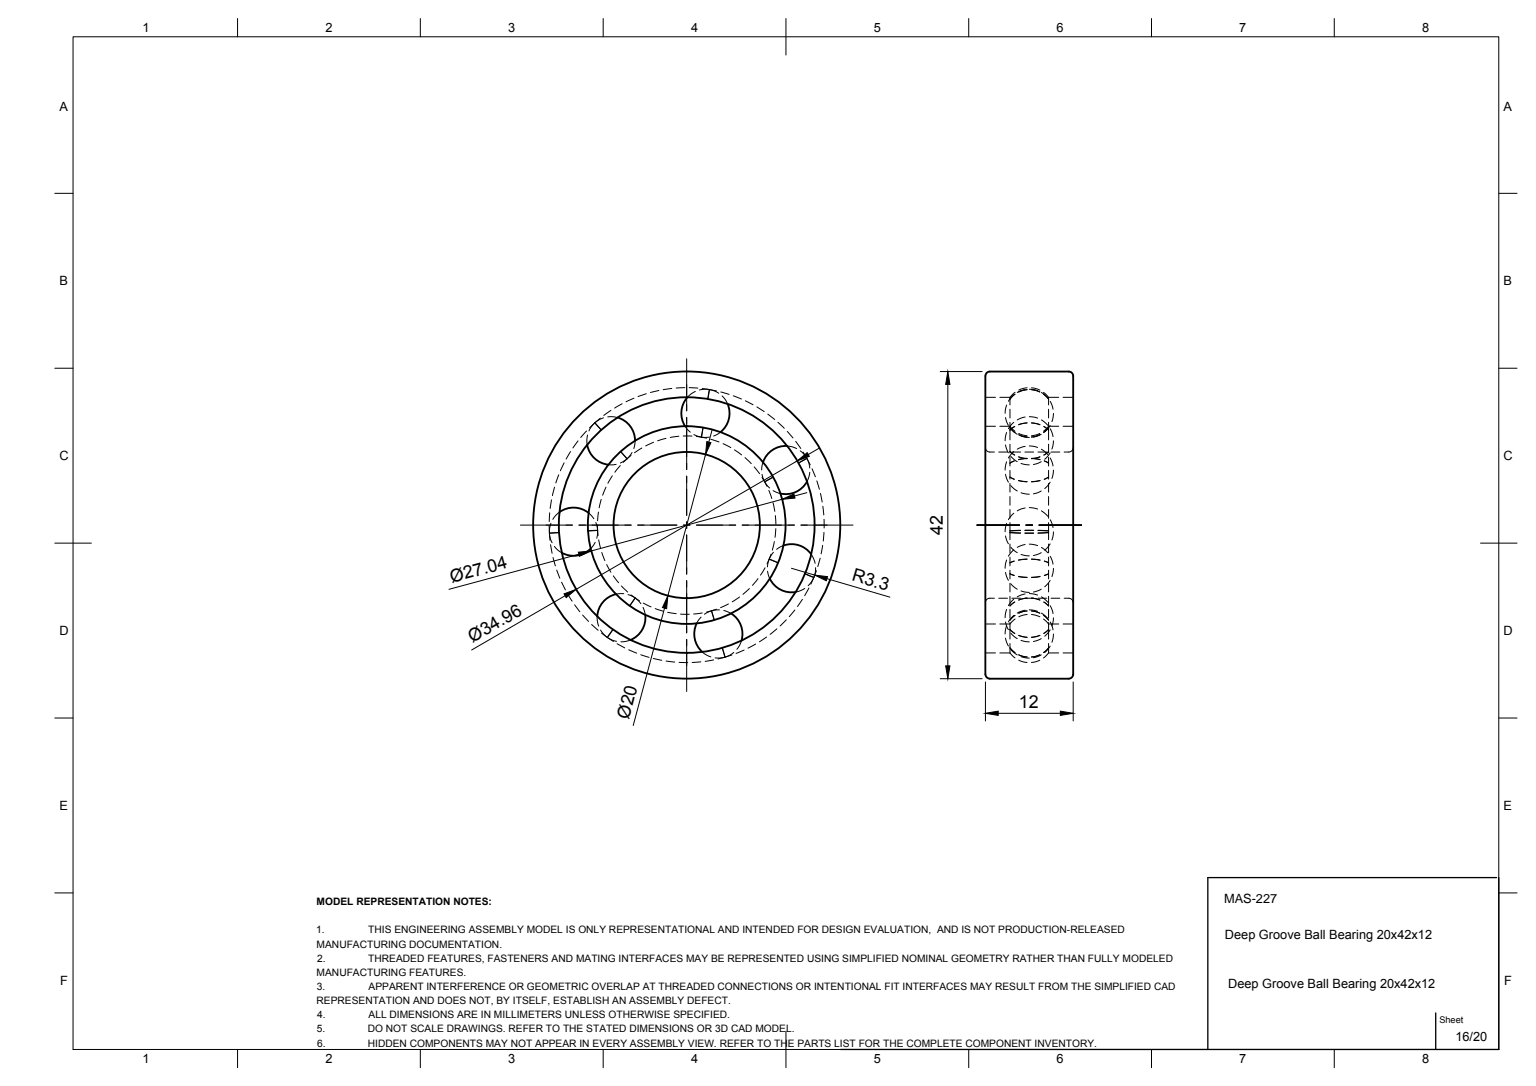
ISO-10303-21;
HEADER;
FILE_DESCRIPTION (('STEP AP214'),
    '1' );
FILE_NAME ( 'Deep Groove Ball Bearing 20x42x12.step', '2026-10-06T08:24:41', ( '' ), ( '' ), 'STEP AP214', 'Unspecified', '' );
FILE_SCHEMA (( 'AUTOMOTIVE_DESIGN' ));
ENDSEC;
DATA;
#17=EDGE_LOOP ( 'NONE', ( #23357, #276 ) ) ;
#28=EDGE_LOOP ( 'NONE', ( #27536, #25941, #6890, #26998 ) ) ;
#30=CARTESIAN_POINT ( 'NONE',  ( -0.5949363243629232079, -0.1357903337134990229, 0.2362204724409449064 ) ) ;
#38=AXIS2_PLACEMENT_3D ( 'NONE', #5001, #26071, #6729 ) ;
#39=CARTESIAN_POINT ( 'NONE',  ( 0.000000000000000000, 0.000000000000000000, 0.06614173228346456601 ) ) ;
#43=CARTESIAN_POINT ( 'NONE',  ( 0.000000000000000000, 0.000000000000000000, 0.2362204724409449064 ) ) ;
#48=ORIENTED_EDGE ( 'NONE', *, *, #8188, .T. ) ;
#58=CARTESIAN_POINT ( 'NONE',  ( 0.4771018889076559244, 0.3804760601893846794, 0.2362204724409449064 ) ) ;
#64=CARTESIAN_POINT ( 'NONE',  ( 0.4157391792961063204, 0.3323952789219082882, 0.1322834645669291320 ) ) ;
#67=CARTESIAN_POINT ( 'NONE',  ( 0.8031496062992127261, 0.000000000000000000, 0.4488188976377953110 ) ) ;
#86=EDGE_CURVE ( 'NONE', #9806, #21006, #24069, .T. ) ;
#87=FACE_BOUND ( 'NONE', #23508, .T. ) ;
#107=ORIENTED_EDGE ( 'NONE', *, *, #20255, .T. ) ;
#109=ADVANCED_FACE ( 'NONE', ( #134 ), #14626, .F. ) ;
#134=FACE_OUTER_BOUND ( 'NONE', #7605, .T. ) ;
#136=CARTESIAN_POINT ( 'NONE',  ( 0.000000000000000000, 0.000000000000000000, 0.2362204724409449064 ) ) ;
#143=CARTESIAN_POINT ( 'NONE',  ( 0.5614173959481695286, 0.4467232815848914962, 0.1601585119481469810 ) ) ;
#153=AXIS2_PLACEMENT_3D ( 'NONE', #12101, #3470, #22847 ) ;
#167=DIRECTION ( 'NONE',  ( 1.000000000000000000, 0.000000000000000000, 0.000000000000000000 ) ) ;
#178=CARTESIAN_POINT ( 'NONE',  ( 0.000000000000000000, 0.000000000000000000, 0.2362204724409449064 ) ) ;
#185=CARTESIAN_POINT ( 'NONE',  ( 0.0007595033562148819414, 0.6881885572739390167, 0.1322834645669291320 ) ) ;
#209=EDGE_CURVE ( 'NONE', #16657, #13154, #17294, .T. ) ;
#219=VECTOR ( 'NONE', #3397, 39.37007874015748143 ) ;
#223=CARTESIAN_POINT ( 'NONE',  ( 0.0005057506112066243896, 0.6881888373222778688, 0.3401591245381555551 ) ) ;
#242=AXIS2_PLACEMENT_3D ( 'NONE', #867, #7637, #22743 ) ;
#257=AXIS2_PLACEMENT_3D ( 'NONE', #24962, #7448, #3195 ) ;
#267=EDGE_CURVE ( 'NONE', #4877, #9806, #20517, .T. ) ;
#269=CARTESIAN_POINT ( 'NONE',  ( 0.3751294191746885609, 0.2999672986753447734, 0.2362204724409446843 ) ) ;
#276=ORIENTED_EDGE ( 'NONE', *, *, #1809, .T. ) ;
#297=CARTESIAN_POINT ( 'NONE',  ( -0.6708219662590964028, -0.1536294932067021612, 0.1322818203437344520 ) ) ;
#299=CARTESIAN_POINT ( 'NONE',  ( -0.5190862322091315262, -0.1177929122753175184, 0.3401574803149606252 ) ) ;
#335=CARTESIAN_POINT ( 'NONE',  ( 0.000000000000000000, 0.000000000000000000, 0.2362204724409449064 ) ) ;
#338=ORIENTED_EDGE ( 'NONE', *, *, #23140, .F. ) ;
#350=CARTESIAN_POINT ( 'NONE',  ( 0.6996455634132897616, -0.1588938903156011662, 0.1601585119484411623 ) ) ;
#389=DIMENSIONAL_EXPONENTS ( 1.000000000000000000, 0.000000000000000000, 0.000000000000000000, 0.000000000000000000, 0.000000000000000000, 0.000000000000000000, 0.000000000000000000 ) ;
#397=B_SPLINE_CURVE_WITH_KNOTS ( 'NONE', 3,
 ( #22454, #26273, #15820, #17525, #20191, #11434, #11714, #3081 ),
 .UNSPECIFIED., .F., .F.,
 ( 4, 2, 2, 4 ),
 ( 0.5000000000000000000, 0.7499999999999997780, 0.8749999999999998890, 1.000000000000000000 ),
 .UNSPECIFIED. ) ;
#401=VERTEX_POINT ( 'NONE', #26015 ) ;
#410=DIRECTION ( 'NONE',  ( 0.000000000000000000, 0.000000000000000000, 1.000000000000000000 ) ) ;
#414=ORIENTED_EDGE ( 'NONE', *, *, #16074, .T. ) ;
#422=CARTESIAN_POINT ( 'NONE',  ( -0.5188388941967637669, -0.1188778293835246053, 0.3401591244667909186 ) ) ;
#423=CIRCLE ( 'NONE', #2649, 0.6881889763779527325 ) ;
#428=ORIENTED_EDGE ( 'NONE', *, *, #19664, .T. ) ;
#432=ORIENTED_EDGE ( 'NONE', *, *, #5914, .T. ) ;
#456=CARTESIAN_POINT ( 'NONE',  ( -0.4684132450478830645, -0.1062614382955276715, 0.2362204724409449619 ) ) ;
#460=CARTESIAN_POINT ( 'NONE',  ( -0.5190862322091315262, -0.1177929122753175184, 0.3401574803149606252 ) ) ;
#462=CARTESIAN_POINT ( 'NONE',  ( 0.4887136534578185310, -0.1122103150229527835, 0.1643955689280507948 ) ) ;
#467=CARTESIAN_POINT ( 'NONE',  ( -0.2981382804007346454, -0.6202561546315846774, 0.1322818203437346463 ) ) ;
#489=CIRCLE ( 'NONE', #20321, 0.5322834645669292097 ) ;
#491=ADVANCED_FACE ( 'NONE', ( #21504 ), #18663, .F. ) ;
#492=FACE_BOUND ( 'NONE', #4958, .T. ) ;
#506=ORIENTED_EDGE ( 'NONE', *, *, #4372, .T. ) ;
#523=EDGE_LOOP ( 'NONE', ( #21704, #21460, #12292, #1622, #7292, #18239 ) ) ;
#531=ORIENTED_EDGE ( 'NONE', *, *, #2877, .F. ) ;
#536=CIRCLE ( 'NONE', #16320, 0.3937007874015748254 ) ;
#543=CARTESIAN_POINT ( 'NONE',  ( -0.0006620872580281702332, 0.5229309616561139684, 0.3331434174598592590 ) ) ;
#548=CARTESIAN_POINT ( 'NONE',  ( 0.0006679551606482677165, 0.5322830454629158270, 0.1322834645669291320 ) ) ;
#554=ORIENTED_EDGE ( 'NONE', *, *, #13765, .T. ) ;
#565=ADVANCED_FACE ( 'NONE', ( #2546 ), #3319, .F. ) ;
#570=CARTESIAN_POINT ( 'NONE',  ( 0.3105958729527036888, -0.6467467715322953170, 0.3122824329341910010 ) ) ;
#577=CARTESIAN_POINT ( 'NONE',  ( 0.000000000000000000, 0.000000000000000000, 0.2362204724409449064 ) ) ;
#598=CARTESIAN_POINT ( 'NONE',  ( 0.6996455634117477729, -0.1588938903152396498, 0.3122824329354899064 ) ) ;
#600=CIRCLE ( 'NONE', #12333, 0.8267716535433071723 ) ;
#618=CARTESIAN_POINT ( 'NONE',  ( -0.0005057506112066828281, 0.6881888373222776467, 0.3401591245381555551 ) ) ;
#619=CARTESIAN_POINT ( 'NONE',  ( 0.2988215684304370012, -0.6199272547993012195, 0.3401599409343967761 ) ) ;
#626=DIRECTION ( 'NONE',  ( 0.000000000000000000, 1.000000000000000000, 0.000000000000000000 ) ) ;
#644=ORIENTED_EDGE ( 'NONE', *, *, #7697, .T. ) ;
#682=SPHERICAL_SURFACE ( 'NONE', #15113, 0.1299232283464566984 ) ;
#695=ORIENTED_EDGE ( 'NONE', *, *, #25428, .F. ) ;
#699=CARTESIAN_POINT ( 'NONE',  ( 0.3759206409296169116, 0.2989751379763687655, 0.2362204724409450174 ) ) ;
#708=FACE_OUTER_BOUND ( 'NONE', #15095, .T. ) ;
#712=DIRECTION ( 'NONE',  ( 0.000000000000000000, -1.000000000000000000, 0.000000000000000000 ) ) ;
#728=CARTESIAN_POINT ( 'NONE',  ( 0.5385210225480960844, 0.4284847435812472183, 0.1322834645669291320 ) ) ;
#739=CARTESIAN_POINT ( 'NONE',  ( 0.000000000000000000, 0.000000000000000000, -1.092739370078740131E-17 ) ) ;
#758=FACE_BOUND ( 'NONE', #21251, .T. ) ;
#768=CARTESIAN_POINT ( 'NONE',  ( 0.0006679551606482677165, 0.5322830454629158270, 0.3401574803149606252 ) ) ;
#793=ORIENTED_EDGE ( 'NONE', *, *, #18272, .F. ) ;
#809=PLANE ( 'NONE',  #6198 ) ;
#819=CARTESIAN_POINT ( 'NONE',  ( -0.2303471512294322787, -0.4798602677570401598, 0.1322834645669291320 ) ) ;
#842=CARTESIAN_POINT ( 'NONE',  ( 0.4092566936341573980, 0.3255244810069335970, 0.3331434174606269227 ) ) ;
#864=CARTESIAN_POINT ( 'NONE',  ( 0.2092582568863658732, -0.4359957531143022202, 0.2715646632236008440 ) ) ;
#867=CARTESIAN_POINT ( 'NONE',  ( 0.000000000000000000, 0.000000000000000000, 0.2362204724409449064 ) ) ;
#874=LINE ( 'NONE', #22052, #17827 ) ;
#883=AXIS2_PLACEMENT_3D ( 'NONE', #21381, #23084, #14476 ) ;
#899=CARTESIAN_POINT ( 'NONE',  ( 0.2315507648392299000, -0.4792806379917101678, 0.1322834645669291320 ) ) ;
#901=EDGE_CURVE ( 'NONE', #11142, #9968, #10681, .T. ) ;
#902=CARTESIAN_POINT ( 'NONE',  ( 0.2307489990847578776, -0.4796672131996535526, 0.1322810039474933141 ) ) ;
#908=ORIENTED_EDGE ( 'NONE', *, *, #10737, .T. ) ;
#910=CARTESIAN_POINT ( 'NONE',  ( 0.4157391792961063204, 0.3323952789219082882, 0.1322834645669291320 ) ) ;
#929=AXIS2_PLACEMENT_3D ( 'NONE', #24250, #9255, #13939 ) ;
#942=ORIENTED_EDGE ( 'NONE', *, *, #7366, .T. ) ;
#956=( GEOMETRIC_REPRESENTATION_CONTEXT ( 3 ) GLOBAL_UNCERTAINTY_ASSIGNED_CONTEXT ( ( #13843 ) ) GLOBAL_UNIT_ASSIGNED_CONTEXT ( ( #21076, #968, #13392 ) ) REPRESENTATION_CONTEXT ( 'NONE', 'WORKASPACE' ) ) ;
#962=CARTESIAN_POINT ( 'NONE',  ( -0.7168072604740280962, -0.1644124225524362104, 0.2763636194370550636 ) ) ;
#967=EDGE_CURVE ( 'NONE', #6542, #17886, #4274, .T. ) ;
#968=( NAMED_UNIT ( * ) PLANE_ANGLE_UNIT ( ) SI_UNIT ( $, .RADIAN. ) ) ;
#972=ORIENTED_EDGE ( 'NONE', *, *, #10601, .F. ) ;
#991=FACE_OUTER_BOUND ( 'NONE', #24406, .T. ) ;
#996=EDGE_LOOP ( 'NONE', ( #23679, #19613, #11944, #25991 ) ) ;
#1016=B_SPLINE_CURVE_WITH_KNOTS ( 'NONE', 3,
 ( #6689, #6828, #4154, #12764, #10638, #19260, #23362, #17146 ),
 .UNSPECIFIED., .F., .F.,
 ( 4, 2, 2, 4 ),
 ( 0.5000000000000000000, 0.7500000000000000000, 0.8749999999999998890, 1.000000000000000000 ),
 .UNSPECIFIED. ) ;
#1017=DIRECTION ( 'NONE',  ( 1.000000000000000000, 0.000000000000000000, 0.000000000000000000 ) ) ;
#1041=DIRECTION ( 'NONE',  ( 0.000000000000000000, -1.000000000000000000, 0.000000000000000000 ) ) ;
#1063=CARTESIAN_POINT ( 'NONE',  ( -0.2274877609455561167, -0.4708572476080006841, 0.1392975274314397494 ) ) ;
#1067=DIRECTION ( 'NONE',  ( -0.2225209339563148925, -0.9749279121818235083, 0.000000000000000000 ) ) ;
#1068=EDGE_CURVE ( 'NONE', #24735, #4219, #15983, .T. ) ;
#1069=EDGE_LOOP ( 'NONE', ( #7141, #12529 ) ) ;
#1077=CARTESIAN_POINT ( 'NONE',  ( 0.4771018889076559244, 0.3804760601893846794, 0.2362204724409449064 ) ) ;
#1094=CARTESIAN_POINT ( 'NONE',  ( 0.000000000000000000, 0.000000000000000000, 0.1322834645669291320 ) ) ;
#1102=AXIS2_PLACEMENT_3D ( 'NONE', #11901, #14175, #1443 ) ;
#1104=CARTESIAN_POINT ( 'NONE',  ( -8.427884271297532088E-17, -0.6881889763779527325, -1.092739370078740131E-17 ) ) ;
#1118=CARTESIAN_POINT ( 'NONE',  ( 0.6708784387195235732, -0.1533826961018693036, 0.3401599409343967761 ) ) ;
#1141=TOROIDAL_SURFACE ( 'NONE', #20078, 0.6102362204724409711, 0.1299212598425196763 ) ;
#1160=ADVANCED_FACE ( 'NONE', ( #25108, #24822 ), #23001, .T. ) ;
#1161=CIRCLE ( 'NONE', #15602, 0.8031496062992127261 ) ;
#1162=ADVANCED_FACE ( 'NONE', ( #9991 ), #18161, .F. ) ;
#1173=CARTESIAN_POINT ( 'NONE',  ( -0.4771018889076559244, 0.3804760601893846794, 0.2362204724409449064 ) ) ;
#1183=DIRECTION ( 'NONE',  ( 0.000000000000000000, 0.000000000000000000, -1.000000000000000000 ) ) ;
#1191=ORIENTED_EDGE ( 'NONE', *, *, #24120, .T. ) ;
#1206=EDGE_LOOP ( 'NONE', ( #20592, #15757, #18634, #4273, #12078, #24003 ) ) ;
#1208=EDGE_CURVE ( 'NONE', #4395, #4877, #8780, .T. ) ;
#1211=DIRECTION ( 'NONE',  ( 1.000000000000000000, 0.000000000000000000, 0.000000000000000000 ) ) ;
#1236=DIRECTION ( 'NONE',  ( 0.000000000000000000, 0.000000000000000000, 1.000000000000000000 ) ) ;
#1237=B_SPLINE_CURVE_WITH_KNOTS ( 'NONE', 3,
 ( #6570, #10655, #1901, #23804, #17029, #25640 ),
 .UNSPECIFIED., .F., .F.,
 ( 4, 2, 4 ),
 ( 1.217380381967464009, 1.219305002860850085, 1.221229623754233939 ),
 .UNSPECIFIED. ) ;
#1243=CARTESIAN_POINT ( 'NONE',  ( -0.7214243740396926174, -0.1654689342655534801, 0.2161412452766471592 ) ) ;
#1261=( GEOMETRIC_REPRESENTATION_CONTEXT ( 3 ) GLOBAL_UNCERTAINTY_ASSIGNED_CONTEXT ( ( #4018 ) ) GLOBAL_UNIT_ASSIGNED_CONTEXT ( ( #20102, #7243, #11487 ) ) REPRESENTATION_CONTEXT ( 'NONE', 'WORKASPACE' ) ) ;
#1281=ORIENTED_EDGE ( 'NONE', *, *, #26449, .F. ) ;
#1291=ORIENTED_EDGE ( 'NONE', *, *, #14066, .F. ) ;
#1300=ORIENTED_EDGE ( 'NONE', *, *, #15873, .F. ) ;
#1307=CARTESIAN_POINT ( 'NONE',  ( -8.427884271297532088E-17, -0.6881889763779527325, 0.06614173228346456601 ) ) ;
#1313=ORIENTED_EDGE ( 'NONE', *, *, #2014, .T. ) ;
#1321=AXIS2_PLACEMENT_3D ( 'NONE', #1328, #3417, #16302 ) ;
#1328=CARTESIAN_POINT ( 'NONE',  ( 0.000000000000000000, 0.000000000000000000, 0.1322834645669291320 ) ) ;
#1334=CARTESIAN_POINT ( 'NONE',  ( -0.4684132450478830645, -0.1062614382955276715, 0.2362204724409449619 ) ) ;
#1347=DIRECTION ( 'NONE',  ( 1.000000000000000000, 0.000000000000000000, 0.000000000000000000 ) ) ;
#1366=EDGE_CURVE ( 'NONE', #18057, #27874, #11501, .T. ) ;
#1385=CARTESIAN_POINT ( 'NONE',  ( 0.2992781133268291316, -0.6197069291944922176, 0.1322834645669291320 ) ) ;
#1386=DIRECTION ( 'NONE',  ( 0.000000000000000000, -1.000000000000000000, 0.000000000000000000 ) ) ;
#1410=EDGE_LOOP ( 'NONE', ( #2496, #1567, #26591, #14884 ) ) ;
#1421=VERTEX_POINT ( 'NONE', #8166 ) ;
#1426=TOROIDAL_SURFACE ( 'NONE', #22181, 0.8031496062992127261, 0.02362204724409448786 ) ;
#1437=CARTESIAN_POINT ( 'NONE',  ( -0.4887136534571460689, -0.1122103150228022234, 0.3080453759528285484 ) ) ;
#1443=DIRECTION ( 'NONE',  ( 0.000000000000000000, 1.000000000000000000, 0.000000000000000000 ) ) ;
#1449=ORIENTED_EDGE ( 'NONE', *, *, #11538, .T. ) ;
#1452=CARTESIAN_POINT ( 'NONE',  ( 0.2078289949484099508, -0.4330237525398077936, 0.2362204724409449619 ) ) ;
#1461=ORIENTED_EDGE ( 'NONE', *, *, #22420, .T. ) ;
#1474=EDGE_CURVE ( 'NONE', #21273, #6542, #24194, .T. ) ;
#1479=CARTESIAN_POINT ( 'NONE',  ( 0.5781866216494347954, 0.4620966632776112304, 0.2562996996002243066 ) ) ;
#1491=ORIENTED_EDGE ( 'NONE', *, *, #6631, .F. ) ;
#1508=TOROIDAL_SURFACE ( 'NONE', #17296, 0.6102362204724409711, 0.1299212598425196763 ) ;
#1515=CARTESIAN_POINT ( 'NONE',  ( 0.000000000000000000, 0.000000000000000000, 0.3401574803149606252 ) ) ;
#1516=AXIS2_PLACEMENT_3D ( 'NONE', #8600, #17220, #167 ) ;
#1523=DIRECTION ( 'NONE',  ( 0.000000000000000000, 0.000000000000000000, 1.000000000000000000 ) ) ;
#1526=EDGE_CURVE ( 'NONE', #23608, #18057, #15118, .T. ) ;
#1527=CARTESIAN_POINT ( 'NONE',  ( 0.000000000000000000, 0.000000000000000000, 0.4062992125984251635 ) ) ;
#1538=EDGE_CURVE ( 'NONE', #8989, #14684, #13758, .T. ) ;
#1539=EDGE_CURVE ( 'NONE', #2213, #9968, #20982, .T. ) ;
#1542=SPHERICAL_SURFACE ( 'NONE', #17946, 0.1299232283464566984 ) ;
#1564=VERTEX_POINT ( 'NONE', #24234 ) ;
#1565=EDGE_CURVE ( 'NONE', #2213, #15981, #2226, .T. ) ;
#1567=ORIENTED_EDGE ( 'NONE', *, *, #26156, .F. ) ;
#1575=CARTESIAN_POINT ( 'NONE',  ( -0.0006679551606482677165, 0.5322830454629158270, 0.3401574803149606252 ) ) ;
#1577=EDGE_LOOP ( 'NONE', ( #3628, #6530 ) ) ;
#1590=CIRCLE ( 'NONE', #2500, 0.02362204724409448092 ) ;
#1608=EDGE_CURVE ( 'NONE', #17836, #10270, #11374, .T. ) ;
#1622=ORIENTED_EDGE ( 'NONE', *, *, #6377, .T. ) ;
#1628=EDGE_CURVE ( 'NONE', #9678, #24310, #22787, .T. ) ;
#1647=B_SPLINE_CURVE_WITH_KNOTS ( 'NONE', 3,
 ( #2295, #10921, #26037, #9470, #11886, #5244 ),
 .UNSPECIFIED., .F., .F.,
 ( 4, 2, 4 ),
 ( 0.4045103800605749922, 0.4064350009536160102, 0.4083596218466570282 ),
 .UNSPECIFIED. ) ;
#1679=DIRECTION ( 'NONE',  ( 0.000000000000000000, 0.000000000000000000, 1.000000000000000000 ) ) ;
#1680=CARTESIAN_POINT ( 'NONE',  ( -0.5385210225480960844, 0.4284847435812472183, 0.1322834645669291320 ) ) ;
#1693=EDGE_CURVE ( 'NONE', #27602, #16511, #21795, .T. ) ;
#1712=CARTESIAN_POINT ( 'NONE',  ( 0.0002221395201541382898, 0.5322834645669292097, 0.1322810039474933141 ) ) ;
#1718=EDGE_CURVE ( 'NONE', #4754, #27858, #20544, .T. ) ;
#1720=EDGE_CURVE ( 'NONE', #27077, #22659, #4736, .T. ) ;
#1730=AXIS2_PLACEMENT_3D ( 'NONE', #1173, #4976, #2977 ) ;
#1732=CIRCLE ( 'NONE', #27448, 0.02362204724409448786 ) ;
#1746=DIRECTION ( 'NONE',  ( 0.000000000000000000, 0.000000000000000000, 1.000000000000000000 ) ) ;
#1755=VERTEX_POINT ( 'NONE', #9920 ) ;
#1762=DIRECTION ( 'NONE',  ( 1.000000000000000000, 0.000000000000000000, 0.000000000000000000 ) ) ;
#1772=AXIS2_PLACEMENT_3D ( 'NONE', #26756, #16030, #5286 ) ;
#1774=AXIS2_PLACEMENT_3D ( 'NONE', #6050, #23287, #16772 ) ;
#1794=AXIS2_PLACEMENT_3D ( 'NONE', #3332, #8026, #8807 ) ;
#1809=EDGE_CURVE ( 'NONE', #18324, #3673, #7442, .T. ) ;
#1814=ORIENTED_EDGE ( 'NONE', *, *, #967, .F. ) ;
#1837=ORIENTED_EDGE ( 'NONE', *, *, #5197, .F. ) ;
#1844=CARTESIAN_POINT ( 'NONE',  ( -0.3062557396300204515, -0.6341756901046630146, 0.1443310008627645136 ) ) ;
#1874=DIRECTION ( 'NONE',  ( 0.6234898018587330393, -0.7818314824680302477, 0.000000000000000000 ) ) ;
#1878=ORIENTED_EDGE ( 'NONE', *, *, #21317, .T. ) ;
#1901=CARTESIAN_POINT ( 'NONE',  ( -0.6708784387195235732, -0.1533826961018689150, 0.3401599409343967761 ) ) ;
#1928=CARTESIAN_POINT ( 'NONE',  ( -0.7171569026305500971, -0.1628805401855070167, 0.2763636194294596948 ) ) ;
#1931=ADVANCED_FACE ( 'NONE', ( #21885, #3056 ), #18165, .T. ) ;
#1942=VERTEX_POINT ( 'NONE', #2521 ) ;
#1963=CARTESIAN_POINT ( 'NONE',  ( -0.6711032387266614441, -0.1523958994813200962, 0.1322834645669291320 ) ) ;
#1971=CLOSED_SHELL ( 'NONE', ( #15948, #15056, #8958, #16202, #10885, #14911, #6900, #2595, #9142, #9759, #11797, #21604, #23526, #3346, #19780, #1160, #17922, #5843, #15313, #9809, #10332, #20220, #565, #12662, #11099, #23134, #1162, #26300, #20891, #109, #23751, #26904, #15516, #491, #12592, #16279, #12320, #22712, #12212, #21149, #4868, #10021, #11378, #13614, #8619, #10786, #4999, #11411, #19167, #7508, #16182, #21953, #18937, #16308, #1931, #10879, #21976, #24048, #23772, #7397, #25804, #17407 ) ) ;
#1974=CARTESIAN_POINT ( 'NONE',  ( 0.3119936278842271316, -0.6460736482368880651, 0.3122824329307916646 ) ) ;
#1978=SPHERICAL_SURFACE ( 'NONE', #5233, 0.1299232283464566984 ) ;
#1997=CARTESIAN_POINT ( 'NONE',  ( 0.000000000000000000, 0.000000000000000000, 0.2362204724409449064 ) ) ;
#2014=EDGE_CURVE ( 'NONE', #22651, #5888, #26397, .T. ) ;
#2016=DIRECTION ( 'NONE',  ( 0.000000000000000000, 0.000000000000000000, -1.000000000000000000 ) ) ;
#2058=AXIS2_PLACEMENT_3D ( 'NONE', #16152, #15733, #24751 ) ;
#2087=ORIENTED_EDGE ( 'NONE', *, *, #5920, .F. ) ;
#2105=CARTESIAN_POINT ( 'NONE',  ( -0.6708784387195275700, -0.1533826961018543433, 0.1322810039474933141 ) ) ;
#2118=CARTESIAN_POINT ( 'NONE',  ( 0.3197948809237959322, -0.6622502000717108706, 0.2763636194327128148 ) ) ;
#2128=CARTESIAN_POINT ( 'NONE',  ( 0.000000000000000000, 0.000000000000000000, -1.092739370078740131E-17 ) ) ;
#2131=CARTESIAN_POINT ( 'NONE',  ( -0.2979095355689177493, -0.6203660015065670663, 0.1322834645669291320 ) ) ;
#2134=CARTESIAN_POINT ( 'NONE',  ( 0.000000000000000000, 0.6881889763779527325, 0.1322810039474933141 ) ) ;
#2167=CARTESIAN_POINT ( 'NONE',  ( 0.000000000000000000, 0.000000000000000000, 0.2362204724409449064 ) ) ;
#2192=CARTESIAN_POINT ( 'NONE',  ( 0.5190862322091315262, -0.1177929122753177127, 0.1322834645669291320 ) ) ;
#2213=VERTEX_POINT ( 'NONE', #10133 ) ;
#2217=AXIS2_PLACEMENT_3D ( 'NONE', #27293, #25163, #7943 ) ;
#2226=B_SPLINE_CURVE_WITH_KNOTS ( 'NONE', 3,
 ( #2337, #9236, #20129, #19859, #23963, #7142 ),
 .UNSPECIFIED., .F., .F.,
 ( 4, 2, 4 ),
 ( 0.3864984308775630262, 0.3881911340211379735, 0.3898838371647110335 ),
 .UNSPECIFIED. ) ;
#2229=EDGE_CURVE ( 'NONE', #17886, #21686, #2935, .T. ) ;
#2231=CARTESIAN_POINT ( 'NONE',  ( 0.3751294191746885609, 0.2999672986753447734, 0.2362204724409446843 ) ) ;
#2245=CARTESIAN_POINT ( 'NONE',  ( 0.4021324607160879361, 0.3215300179764621347, 0.1473214333187666258 ) ) ;
#2252=FACE_OUTER_BOUND ( 'NONE', #17, .T. ) ;
#2265=CARTESIAN_POINT ( 'NONE',  ( 0.000000000000000000, 0.6881889763779527325, -1.092739370078740131E-17 ) ) ;
#2268=EDGE_CURVE ( 'NONE', #11692, #16657, #22347, .T. ) ;
#2279=STYLED_ITEM ( 'NONE', ( #12321 ), #12108 ) ;
#2280=ORIENTED_EDGE ( 'NONE', *, *, #17574, .F. ) ;
#2281=VERTEX_POINT ( 'NONE', #23539 ) ;
#2295=CARTESIAN_POINT ( 'NONE',  ( 0.2979095355690402069, -0.6203660015065080024, 0.1322834645669291320 ) ) ;
#2303=CARTESIAN_POINT ( 'NONE',  ( -0.5744851493209846005, 0.4591414886187322741, 0.2763636194302094284 ) ) ;
#2308=B_SPLINE_CURVE_WITH_KNOTS ( 'NONE', 3,
 ( #2134, #4396, #25868, #14201 ),
 .UNSPECIFIED., .F., .F.,
 ( 4, 4 ),
 ( 0.4064350009536160102, 0.4083596218470010308 ),
 .UNSPECIFIED. ) ;
#2312=CARTESIAN_POINT ( 'NONE',  ( -0.2979095355689177493, -0.6203660015065670663, 0.3401574803149606252 ) ) ;
#2337=CARTESIAN_POINT ( 'NONE',  ( -0.4165721057576322606, 0.3313508221749649763, 0.1322834645669291320 ) ) ;
#2364=EDGE_LOOP ( 'NONE', ( #4572, #27619 ) ) ;
#2368=CARTESIAN_POINT ( 'NONE',  ( -0.0006443779181928191001, 0.4960456921223007076, 0.2989974301413287905 ) ) ;
#2386=DIRECTION ( 'NONE',  ( -0.4338837391175582869, -0.9009688679024190350, 0.000000000000000000 ) ) ;
#2388=EDGE_CURVE ( 'NONE', #23587, #2742, #1237, .T. ) ;
#2389=EDGE_CURVE ( 'NONE', #15780, #16922, #8394, .T. ) ;
#2400=CARTESIAN_POINT ( 'NONE',  ( 0.6708784387195275700, -0.1533826961018547319, 0.1322810039474933141 ) ) ;
#2431=FACE_OUTER_BOUND ( 'NONE', #12256, .T. ) ;
#2444=CARTESIAN_POINT ( 'NONE',  ( -0.0006345105826668660581, 0.4803145415259079121, 0.2362204724409446843 ) ) ;
#2453=DIRECTION ( 'NONE',  ( 0.000000000000000000, 0.000000000000000000, 1.000000000000000000 ) ) ;
#2481=CARTESIAN_POINT ( 'NONE',  ( 0.4837521785366984406, -0.1097523286760182931, 0.2989974301281582147 ) ) ;
#2485=EDGE_CURVE ( 'NONE', #8723, #3886, #9728, .T. ) ;
#2496=ORIENTED_EDGE ( 'NONE', *, *, #9868, .F. ) ;
#2498=AXIS2_PLACEMENT_3D ( 'NONE', #8653, #4425, #26293 ) ;
#2500=AXIS2_PLACEMENT_3D ( 'NONE', #67, #6248, #14886 ) ;
#2511=DIRECTION ( 'NONE',  ( 0.000000000000000000, 1.000000000000000000, 0.000000000000000000 ) ) ;
#2521=CARTESIAN_POINT ( 'NONE',  ( -0.5375739373539409893, 0.4296723508511047229, 0.3401574803149606252 ) ) ;
#2524=EDGE_LOOP ( 'NONE', ( #17900, #13744 ) ) ;
#2533=CARTESIAN_POINT ( 'NONE',  ( 0.000000000000000000, 0.000000000000000000, 0.4488188976377953110 ) ) ;
#2538=CARTESIAN_POINT ( 'NONE',  ( 0.3048711895203580768, -0.6348424542976517371, 0.3281099440179709448 ) ) ;
#2541=DIRECTION ( 'NONE',  ( 0.000000000000000000, 0.000000000000000000, 1.000000000000000000 ) ) ;
#2546=FACE_OUTER_BOUND ( 'NONE', #22789, .T. ) ;
#2556=SPHERICAL_SURFACE ( 'NONE', #2498, 0.1299232283464566984 ) ;
#2571=DIRECTION ( 'NONE',  ( 0.000000000000000000, 0.000000000000000000, 1.000000000000000000 ) ) ;
#2572=AXIS2_PLACEMENT_3D ( 'NONE', #1077, #5152, #10509 ) ;
#2586=CIRCLE ( 'NONE', #7558, 0.6881889763779527325 ) ;
#2595=ADVANCED_FACE ( 'NONE', ( #26012 ), #4331, .F. ) ;
#2627=ORIENTED_EDGE ( 'NONE', *, *, #4655, .T. ) ;
#2631=CARTESIAN_POINT ( 'NONE',  ( -0.6707652279343464530, -0.1538768215239710857, 0.1322834645669291320 ) ) ;
#2649=AXIS2_PLACEMENT_3D ( 'NONE', #1515, #3620, #10126 ) ;
#2657=CARTESIAN_POINT ( 'NONE',  ( 0.3751294191746888940, 0.2999672986753446624, 0.2194422276300426189 ) ) ;
#2661=CARTESIAN_POINT ( 'NONE',  ( 0.6864238947237005783, -0.1574599019770832331, 0.3281099440179374715 ) ) ;
#2662=EDGE_LOOP ( 'NONE', ( #10373, #24245, #4890, #12960, #14300, #21059 ) ) ;
#2669=CARTESIAN_POINT ( 'NONE',  ( 0.2274877609439496517, -0.4708572476046440358, 0.3331434174476592402 ) ) ;
#2679=CARTESIAN_POINT ( 'NONE',  ( 0.2146455952155474356, -0.4472013107345719218, 0.2989974300902882298 ) ) ;
#2682=CARTESIAN_POINT ( 'NONE',  ( -0.4887136534522864562, -0.1122103150216818279, 0.1643955689363730821 ) ) ;
#2714=CARTESIAN_POINT ( 'NONE',  ( 0.2305483297598421022, -0.4797636960996590760, 0.1322818204150988386 ) ) ;
#2734=CARTESIAN_POINT ( 'NONE',  ( 0.5949363243629232079, -0.1357903337134992172, 0.2362204724409449064 ) ) ;
#2742=VERTEX_POINT ( 'NONE', #10957 ) ;
#2749=FACE_OUTER_BOUND ( 'NONE', #15667, .T. ) ;
#2751=CARTESIAN_POINT ( 'NONE',  ( 0.5021077788561401078, -0.1139291307083168392, 0.1473214333284243727 ) ) ;
#2752=EDGE_CURVE ( 'NONE', #16609, #27306, #2586, .T. ) ;
#2771=CARTESIAN_POINT ( 'NONE',  ( 0.6707652279343347956, -0.1538768215240155779, 0.3401574803149606252 ) ) ;
#2788=CARTESIAN_POINT ( 'NONE',  ( -0.2647715730835492609, -0.5498038367121063086, 0.1062972440944881941 ) ) ;
#2795=CARTESIAN_POINT ( 'NONE',  ( 0.000000000000000000, 0.000000000000000000, 0.3401574803149606252 ) ) ;
#2807=DIRECTION ( 'NONE',  ( 0.000000000000000000, 0.000000000000000000, 1.000000000000000000 ) ) ;
#2831=EDGE_LOOP ( 'NONE', ( #11493, #11739, #18792, #21781 ) ) ;
#2854=VERTEX_POINT ( 'NONE', #11783 ) ;
#2877=EDGE_CURVE ( 'NONE', #2281, #2854, #18362, .T. ) ;
#2881=CARTESIAN_POINT ( 'NONE',  ( -0.4157391792961063204, 0.3323952789219086768, 0.3401574803149606252 ) ) ;
#2889=DIRECTION ( 'NONE',  ( 0.000000000000000000, 0.000000000000000000, 1.000000000000000000 ) ) ;
#2900=CARTESIAN_POINT ( 'NONE',  ( 0.2303471512294322787, -0.4798602677570401598, 0.3401574803149606252 ) ) ;
#2915=DIRECTION ( 'NONE',  ( 0.000000000000000000, 1.000000000000000000, 0.000000000000000000 ) ) ;
#2922=VERTEX_POINT ( 'NONE', #11640 ) ;
#2935=CIRCLE ( 'NONE', #13318, 0.4803149606299212393 ) ;
#2937=DIRECTION ( 'NONE',  ( 0.000000000000000000, 0.000000000000000000, 1.000000000000000000 ) ) ;
#2940=FACE_OUTER_BOUND ( 'NONE', #4320, .T. ) ;
#2946=TOROIDAL_SURFACE ( 'NONE', #18286, 0.6102362204724409711, 0.1299212598425196763 ) ;
#2959=CIRCLE ( 'NONE', #13813, 0.6881889763779527325 ) ;
#2977=DIRECTION ( 'NONE',  ( 0.6234898018587335944, 0.7818314824680296926, 0.000000000000000000 ) ) ;
#2983=LINE ( 'NONE', #6775, #17603 ) ;
#2989=DIRECTION ( 'NONE',  ( 0.000000000000000000, 1.000000000000000000, 0.000000000000000000 ) ) ;
#2992=ORIENTED_EDGE ( 'NONE', *, *, #6972, .T. ) ;
#3035=DIRECTION ( 'NONE',  ( 1.000000000000000000, 0.000000000000000000, 0.000000000000000000 ) ) ;
#3051=CARTESIAN_POINT ( 'NONE',  ( 0.000000000000000000, 0.000000000000000000, 0.4488188976377953110 ) ) ;
#3056=FACE_OUTER_BOUND ( 'NONE', #16842, .T. ) ;
#3063=ORIENTED_EDGE ( 'NONE', *, *, #15128, .T. ) ;
#3081=CARTESIAN_POINT ( 'NONE',  ( -0.4157391792961063204, 0.3323952789219086768, 0.3401574803149606252 ) ) ;
#3088=CARTESIAN_POINT ( 'NONE',  ( 0.0007595033562148819414, 0.6881885572739390167, 0.1322834645669291320 ) ) ;
#3121=CARTESIAN_POINT ( 'NONE',  ( -0.4681308612729627172, -0.1074986424507606841, 0.2362204724409447676 ) ) ;
#3142=CARTESIAN_POINT ( 'NONE',  ( 0.0006443779181925812262, 0.4960456921221567672, 0.2989974301410669444 ) ) ;
#3149=CARTESIAN_POINT ( 'NONE',  ( -0.6711032387266614441, -0.1523958994813200962, 0.1322834645669291320 ) ) ;
#3153=VERTEX_POINT ( 'NONE', #3149 ) ;
#3185=CARTESIAN_POINT ( 'NONE',  ( -1.012503259137575512E-16, -0.8267716535433071723, 0.02362204724409448786 ) ) ;
#3188=CARTESIAN_POINT ( 'NONE',  ( 0.000000000000000000, 0.000000000000000000, 0.2362204724409449064 ) ) ;
#3191=CARTESIAN_POINT ( 'NONE',  ( -0.6993003464547263848, -0.1604063846365767210, 0.3122824329331324034 ) ) ;
#3195=DIRECTION ( 'NONE',  ( 0.000000000000000000, 1.000000000000000000, 0.000000000000000000 ) ) ;
#3199=EDGE_LOOP ( 'NONE', ( #18507, #7887, #23739, #14230, #25167, #506, #9319, #4343, #12090, #12890, #24965, #10457 ) ) ;
#3222=ORIENTED_EDGE ( 'NONE', *, *, #18065, .T. ) ;
#3226=CARTESIAN_POINT ( 'NONE',  ( -0.3916295560419718602, 0.3131429078191630411, 0.1643955689142584109 ) ) ;
#3252=AXIS2_PLACEMENT_3D ( 'NONE', #5989, #19250, #27453 ) ;
#3279=ORIENTED_EDGE ( 'NONE', *, *, #10114, .F. ) ;
#3306=ORIENTED_EDGE ( 'NONE', *, *, #13358, .T. ) ;
#3310=ORIENTED_EDGE ( 'NONE', *, *, #2485, .T. ) ;
#3313=ORIENTED_EDGE ( 'NONE', *, *, #20255, .F. ) ;
#3319=TOROIDAL_SURFACE ( 'NONE', #4680, 0.6102362204724409711, 0.1299212598425196763 ) ;
#3332=CARTESIAN_POINT ( 'NONE',  ( 0.000000000000000000, 0.000000000000000000, -1.092739370078740131E-17 ) ) ;
#3341=DIRECTION ( 'NONE',  ( 1.000000000000000000, 0.000000000000000000, 0.000000000000000000 ) ) ;
#3346=ADVANCED_FACE ( 'NONE', ( #23521 ), #7581, .T. ) ;
#3371=VERTEX_POINT ( 'NONE', #7973 ) ;
#3378=EDGE_CURVE ( 'NONE', #23608, #401, #8941, .T. ) ;
#3384=CIRCLE ( 'NONE', #22817, 0.4173228346456693272 ) ;
#3393=CARTESIAN_POINT ( 'NONE',  ( -0.4681308612729632168, -0.1074986424507606286, 0.2529987172304648535 ) ) ;
#3397=DIRECTION ( 'NONE',  ( 0.000000000000000000, 0.000000000000000000, 1.000000000000000000 ) ) ;
#3417=DIRECTION ( 'NONE',  ( 0.000000000000000000, 0.000000000000000000, 1.000000000000000000 ) ) ;
#3435=B_SPLINE_CURVE_WITH_KNOTS ( 'NONE', 3,
 ( #456, #17538, #19667, #13564, #9175, #13297, #26152, #6808 ),
 .UNSPECIFIED., .F., .F.,
 ( 4, 2, 2, 4 ),
 ( 0.5000000000000000000, 0.7500000000000002220, 0.8750000000000000000, 1.000000000000000000 ),
 .UNSPECIFIED. ) ;
#3444=AXIS2_PLACEMENT_3D ( 'NONE', #18198, #13847, #5077 ) ;
#3455=CARTESIAN_POINT ( 'NONE',  ( -0.8031496062992127261, 9.835745945907876618E-17, 0.4488188976377953110 ) ) ;
#3456=ORIENTED_EDGE ( 'NONE', *, *, #12071, .T. ) ;
#3461=ORIENTED_EDGE ( 'NONE', *, *, #9918, .F. ) ;
#3470=DIRECTION ( 'NONE',  ( 0.000000000000000000, 0.000000000000000000, -1.000000000000000000 ) ) ;
#3488=CARTESIAN_POINT ( 'NONE',  ( -0.8267716535433071723, 1.012503259137575512E-16, 0.02362204724409448786 ) ) ;
#3510=AXIS2_PLACEMENT_3D ( 'NONE', #1997, #26146, #7168 ) ;
#3514=CARTESIAN_POINT ( 'NONE',  ( -0.4157391792961063204, 0.3323952789219086768, 0.1322834645669291320 ) ) ;
#3519=ORIENTED_EDGE ( 'NONE', *, *, #26581, .T. ) ;
#3557=ORIENTED_EDGE ( 'NONE', *, *, #5572, .T. ) ;
#3564=CIRCLE ( 'NONE', #22995, 0.1299212598425196763 ) ;
#3566=CIRCLE ( 'NONE', #1794, 0.5322834645669292097 ) ;
#3569=CARTESIAN_POINT ( 'NONE',  ( -0.0006479495459704965547, 0.5014297259264257622, 0.1643955689169025458 ) ) ;
#3571=ORIENTED_EDGE ( 'NONE', *, *, #27347, .F. ) ;
#3582=CARTESIAN_POINT ( 'NONE',  ( 0.5375739373539409893, 0.4296723508511047229, 0.1322834645669291320 ) ) ;
#3583=CARTESIAN_POINT ( 'NONE',  ( 0.000000000000000000, 0.000000000000000000, 0.2362204724409449064 ) ) ;
#3602=ORIENTED_EDGE ( 'NONE', *, *, #13300, .F. ) ;
#3604=DIRECTION ( 'NONE',  ( 0.000000000000000000, 0.000000000000000000, -1.000000000000000000 ) ) ;
#3620=DIRECTION ( 'NONE',  ( 0.000000000000000000, 0.000000000000000000, 1.000000000000000000 ) ) ;
#3628=ORIENTED_EDGE ( 'NONE', *, *, #22714, .F. ) ;
#3639=ORIENTED_EDGE ( 'NONE', *, *, #26581, .F. ) ;
#3661=AXIS2_PLACEMENT_3D ( 'NONE', #3583, #25070, #5734 ) ;
#3665=DIRECTION ( 'NONE',  ( 0.000000000000000000, 0.000000000000000000, 1.000000000000000000 ) ) ;
#3667=ORIENTED_EDGE ( 'NONE', *, *, #3806, .F. ) ;
#3673=VERTEX_POINT ( 'NONE', #11196 ) ;
#3674=EDGE_CURVE ( 'NONE', #9013, #16391, #17932, .T. ) ;
#3682=CARTESIAN_POINT ( 'NONE',  ( 0.0004447986960614786845, 0.5322833254990984031, 0.1322818204150988386 ) ) ;
#3696=DIRECTION ( 'NONE',  ( 0.000000000000000000, 1.000000000000000000, 0.000000000000000000 ) ) ;
#3701=B_SPLINE_CURVE_WITH_KNOTS ( 'NONE', 3,
 ( #3743, #12363, #18560, #12507, #5742, #10230, #22971, #27207 ),
 .UNSPECIFIED., .F., .F.,
 ( 4, 2, 2, 4 ),
 ( 0.000000000000000000, 0.1249999999999998890, 0.2499999999999997780, 0.5000000000000000000 ),
 .UNSPECIFIED. ) ;
#3708=CARTESIAN_POINT ( 'NONE',  ( -0.0007683673430013719316, 0.7042519390026829029, 0.1443310008634866026 ) ) ;
#3711=CARTESIAN_POINT ( 'NONE',  ( -0.6867658503580778007, -0.1559616964373211900, 0.1443310008614889506 ) ) ;
#3720=CARTESIAN_POINT ( 'NONE',  ( 0.000000000000000000, 0.000000000000000000, 0.3401574803149606252 ) ) ;
#3740=AXIS2_PLACEMENT_3D ( 'NONE', #25412, #21969, #10955 ) ;
#3743=CARTESIAN_POINT ( 'NONE',  ( 0.2303471512294322787, -0.4798602677570401598, 0.1322834645669291320 ) ) ;
#3767=ORIENTED_EDGE ( 'NONE', *, *, #18502, .T. ) ;
#3806=EDGE_CURVE ( 'NONE', #11937, #15780, #19364, .T. ) ;
#3822=CARTESIAN_POINT ( 'NONE',  ( -0.3197948809220744204, -0.6622502000681186329, 0.1960773254378390396 ) ) ;
#3848=DIRECTION ( 'NONE',  ( 0.000000000000000000, 0.000000000000000000, 1.000000000000000000 ) ) ;
#3851=AXIS2_PLACEMENT_3D ( 'NONE', #11182, #4553, #19804 ) ;
#3864=CARTESIAN_POINT ( 'NONE',  ( 0.000000000000000000, 0.8267716535433071723, 0.02362204724409448786 ) ) ;
#3886=VERTEX_POINT ( 'NONE', #14385 ) ;
#3894=DIRECTION ( 'NONE',  ( 0.000000000000000000, 1.000000000000000000, 0.000000000000000000 ) ) ;
#3941=CIRCLE ( 'NONE', #9798, 0.6881889763779527325 ) ;
#3968=EDGE_CURVE ( 'NONE', #27306, #16609, #24749, .T. ) ;
#3970=CARTESIAN_POINT ( 'NONE',  ( -0.2992781133269515892, -0.6197069291944330427, 0.1322834645669291320 ) ) ;
#3972=EDGE_LOOP ( 'NONE', ( #24758, #13354 ) ) ;
#3975=CARTESIAN_POINT ( 'NONE',  ( 0.5383630292499967940, 0.4286833100733393742, 0.3401591245381551110 ) ) ;
#3994=SURFACE_STYLE_USAGE ( .BOTH. , #27444 ) ;
#4018=UNCERTAINTY_MEASURE_WITH_UNIT (LENGTH_MEASURE( 1.000000000000000082E-05 ), #20102, 'distance_accuracy_value', 'NONE') ;
#4031=CARTESIAN_POINT ( 'NONE',  ( 0.000000000000000000, 0.000000000000000000, 0.02362204724409448786 ) ) ;
#4043=CARTESIAN_POINT ( 'NONE',  ( 0.000000000000000000, 0.000000000000000000, 0.3401574803149606252 ) ) ;
#4066=EDGE_CURVE ( 'NONE', #4877, #4395, #23440, .T. ) ;
#4090=TOROIDAL_SURFACE ( 'NONE', #16724, 0.4173228346456693272, 0.02362204724409448786 ) ;
#4114=CARTESIAN_POINT ( 'NONE',  ( 0.5322834645669292097, 0.000000000000000000, 0.1322834645669291320 ) ) ;
#4140=CARTESIAN_POINT ( 'NONE',  ( -0.0004447986960614348285, 0.5322833254990984031, 0.1322818204150988386 ) ) ;
#4150=EDGE_LOOP ( 'NONE', ( #19953, #1191, #3667, #20828, #7453, #14471, #17853, #5870, #22574, #23612, #10773 ) ) ;
#4154=CARTESIAN_POINT ( 'NONE',  ( -0.2092582568885065775, -0.4359957531186999247, 0.2008762816407658747 ) ) ;
#4155=EDGE_CURVE ( 'NONE', #11937, #2922, #6286, .T. ) ;
#4163=EDGE_LOOP ( 'NONE', ( #9471, #7764, #4924, #22930 ) ) ;
#4166=CARTESIAN_POINT ( 'NONE',  ( 0.000000000000000000, 0.6102362204724409711, 0.2362204724409449064 ) ) ;
#4175=EDGE_LOOP ( 'NONE', ( #5300, #5732, #25546, #3767, #11176, #16118, #17476, #16891, #14954, #9551, #27254, #17055 ) ) ;
#4194=CARTESIAN_POINT ( 'NONE',  ( -0.6867658503640922119, -0.1559616964386716931, 0.3281099440157777547 ) ) ;
#4196=ORIENTED_EDGE ( 'NONE', *, *, #17233, .F. ) ;
#4197=CARTESIAN_POINT ( 'NONE',  ( 0.5382052855068000241, 0.4288813374988101890, 0.1322810039474933141 ) ) ;
#4206=AXIS2_PLACEMENT_3D ( 'NONE', #577, #9172, #11438 ) ;
#4219=VERTEX_POINT ( 'NONE', #7445 ) ;
#4232=DIRECTION ( 'NONE',  ( 0.000000000000000000, 0.000000000000000000, 1.000000000000000000 ) ) ;
#4254=DIRECTION ( 'NONE',  ( 0.000000000000000000, 0.000000000000000000, -1.000000000000000000 ) ) ;
#4255=CARTESIAN_POINT ( 'NONE',  ( 0.6102362204724409711, 0.000000000000000000, 0.2362204724409449064 ) ) ;
#4262=CARTESIAN_POINT ( 'NONE',  ( 0.6710470464557933834, -0.1526433524318244195, 0.1322818203437344520 ) ) ;
#4273=ORIENTED_EDGE ( 'NONE', *, *, #1693, .F. ) ;
#4274=CIRCLE ( 'NONE', #6533, 0.4803149606299212393 ) ;
#4280=CARTESIAN_POINT ( 'NONE',  ( 0.5096726623840774906, -0.1170085733297229341, 0.1392975274247515161 ) ) ;
#4292=FACE_OUTER_BOUND ( 'NONE', #11102, .T. ) ;
#4301=DIRECTION ( 'NONE',  ( 0.000000000000000000, 1.000000000000000000, 0.000000000000000000 ) ) ;
#4307=EDGE_CURVE ( 'NONE', #15542, #3371, #12553, .T. ) ;
#4309=DIRECTION ( 'NONE',  ( 0.000000000000000000, -1.000000000000000000, 0.000000000000000000 ) ) ;
#4315=B_SPLINE_CURVE_WITH_KNOTS ( 'NONE', 3,
 ( #7359, #26556, #15979, #24582, #5955, #7645, #3822, #20917, #1844, #3970 ),
 .UNSPECIFIED., .F., .F.,
 ( 4, 2, 2, 2, 4 ),
 ( 0.000000000000000000, 0.2500000000000002776, 0.5000000000000001110, 0.7500000000000000000, 1.000000000000000000 ),
 .UNSPECIFIED. ) ;
#4320=EDGE_LOOP ( 'NONE', ( #554, #5455, #23514, #17998, #19948 ) ) ;
#4323=AXIS2_PLACEMENT_3D ( 'NONE', #11732, #15831, #24581 ) ;
#4331=TOROIDAL_SURFACE ( 'NONE', #20105, 0.6102362204724409711, 0.1299212598425196763 ) ;
#4343=ORIENTED_EDGE ( 'NONE', *, *, #15925, .T. ) ;
#4352=ORIENTED_EDGE ( 'NONE', *, *, #4155, .F. ) ;
#4356=VERTEX_POINT ( 'NONE', #16980 ) ;
#4359=B_SPLINE_CURVE_WITH_KNOTS ( 'NONE', 3,
 ( #24110, #8853, #15642, #7020, #26355, #2751, #19735, #20282 ),
 .UNSPECIFIED., .F., .F.,
 ( 4, 2, 2, 4 ),
 ( 0.5000000000000000000, 0.7500000000000002220, 0.8750000000000000000, 1.000000000000000000 ),
 .UNSPECIFIED. ) ;
#4368=AXIS2_PLACEMENT_3D ( 'NONE', #9283, #2386, #11147 ) ;
#4372=EDGE_CURVE ( 'NONE', #7546, #21258, #22778, .T. ) ;
#4380=FACE_BOUND ( 'NONE', #20747, .T. ) ;
#4395=VERTEX_POINT ( 'NONE', #2265 ) ;
#4396=CARTESIAN_POINT ( 'NONE',  ( -0.0002525749203917322682, 0.6881889763779527325, 0.1322810039474933141 ) ) ;
#4415=ORIENTED_EDGE ( 'NONE', *, *, #10585, .F. ) ;
#4425=DIRECTION ( 'NONE',  ( 0.9749279121818236193, -0.2225209339563147815, 0.000000000000000000 ) ) ;
#4426=ORIENTED_EDGE ( 'NONE', *, *, #18669, .F. ) ;
#4427=CARTESIAN_POINT ( 'NONE',  ( -0.2979095355689177493, -0.6203660015065670663, 0.1322834645669291320 ) ) ;
#4444=CIRCLE ( 'NONE', #3510, 0.4803149606299212393 ) ;
#4446=CARTESIAN_POINT ( 'NONE',  ( -0.0007595033562148819414, 0.6881885572739390167, 0.3401574803149606252 ) ) ;
#4449=DIRECTION ( 'NONE',  ( 0.000000000000000000, 1.000000000000000000, 0.000000000000000000 ) ) ;
#4464=CARTESIAN_POINT ( 'NONE',  ( 0.4684132450478833976, -0.1062614382955264641, 0.2362204724409446843 ) ) ;
#4477=CARTESIAN_POINT ( 'NONE',  ( 0.3874223757879868280, 0.3097832252409934428, 0.2989974301521946543 ) ) ;
#4484=CARTESIAN_POINT ( 'NONE',  ( 0.5510854067038989390, 0.4384931681285572647, 0.3281099440183985472 ) ) ;
#4491=ORIENTED_EDGE ( 'NONE', *, *, #1366, .F. ) ;
#4492=VERTEX_POINT ( 'NONE', #23928 ) ;
#4507=EDGE_CURVE ( 'NONE', #3886, #11422, #11667, .T. ) ;
#4509=EDGE_CURVE ( 'NONE', #17836, #7391, #5385, .T. ) ;
#4517=DIRECTION ( 'NONE',  ( 0.000000000000000000, 0.000000000000000000, 1.000000000000000000 ) ) ;
#4525=CARTESIAN_POINT ( 'NONE',  ( -0.4092566936344115835, 0.3255244810071337702, 0.1392975274210202508 ) ) ;
#4533=CARTESIAN_POINT ( 'NONE',  ( 0.2979095355689177493, -0.6203660015065670663, 0.3401574803149606252 ) ) ;
#4551=CARTESIAN_POINT ( 'NONE',  ( 0.4713455951423065060, -0.1082342125229984742, 0.2008762816149500807 ) ) ;
#4553=DIRECTION ( 'NONE',  ( 0.000000000000000000, 0.000000000000000000, 1.000000000000000000 ) ) ;
#4572=ORIENTED_EDGE ( 'NONE', *, *, #1208, .T. ) ;
#4575=CARTESIAN_POINT ( 'NONE',  ( 0.000000000000000000, 0.000000000000000000, 0.1322834645669291320 ) ) ;
#4587=CARTESIAN_POINT ( 'NONE',  ( 0.000000000000000000, 0.5322834645669292097, 0.4724409448818898127 ) ) ;
#4619=DIRECTION ( 'NONE',  ( -0.2225209339563143096, 0.9749279121818235083, 0.000000000000000000 ) ) ;
#4624=ORIENTED_EDGE ( 'NONE', *, *, #6538, .F. ) ;
#4627=CYLINDRICAL_SURFACE ( 'NONE', #17309, 0.5322834645669292097 ) ;
#4631=FACE_OUTER_BOUND ( 'NONE', #27267, .T. ) ;
#4632=FILL_AREA_STYLE ('',( #11005 ) ) ;
#4637=CARTESIAN_POINT ( 'NONE',  ( 0.3916295560431587996, 0.3131429078201153904, 0.1643955689120278618 ) ) ;
#4645=CARTESIAN_POINT ( 'NONE',  ( 0.6707652279343464530, -0.1538768215239712522, 0.1322834645669291320 ) ) ;
#4655=EDGE_CURVE ( 'NONE', #25431, #17836, #23895, .T. ) ;
#4660=CARTESIAN_POINT ( 'NONE',  ( 0.3204319178469888230, -0.6672004808833374989, 0.2161412452789004401 ) ) ;
#4675=DIRECTION ( 'NONE',  ( 0.000000000000000000, 0.000000000000000000, -1.000000000000000000 ) ) ;
#4680=AXIS2_PLACEMENT_3D ( 'NONE', #26546, #2807, #9308 ) ;
#4689=ORIENTED_EDGE ( 'NONE', *, *, #1718, .T. ) ;
#4696=CARTESIAN_POINT ( 'NONE',  ( -0.5791695622062364990, 0.4608640948057729503, 0.2562996995975141967 ) ) ;
#4703=CARTESIAN_POINT ( 'NONE',  ( -6.518592411209533944E-17, -0.5322834645669292097, -1.092739370078740131E-17 ) ) ;
#4719=AXIS2_PLACEMENT_3D ( 'NONE', #7600, #9709, #5622 ) ;
#4720=CARTESIAN_POINT ( 'NONE',  ( -0.2262947209311158003, -0.4714317853986079720, 0.3331434174507413304 ) ) ;
#4732=CARTESIAN_POINT ( 'NONE',  ( -6.518592411209533944E-17, -0.5322834645669292097, 0.4062992125984251635 ) ) ;
#4736=CIRCLE ( 'NONE', #16024, 0.1299232283464567539 ) ;
#4740=CARTESIAN_POINT ( 'NONE',  ( 0.5385210225480960844, 0.4284847435812472183, 0.3401574803149606252 ) ) ;
#4754=VERTEX_POINT ( 'NONE', #19373 ) ;
#4765=CARTESIAN_POINT ( 'NONE',  ( -0.0006679551606482677165, 0.5322830454629158270, 0.3401574803149606252 ) ) ;
#4792=CARTESIAN_POINT ( 'NONE',  ( 0.3105958729525251649, -0.6467467715319020760, 0.1601585119471421181 ) ) ;
#4803=CARTESIAN_POINT ( 'NONE',  ( 0.2303471512294322787, -0.4798602677570401598, 0.3401574803149606252 ) ) ;
#4808=EDGE_CURVE ( 'NONE', #23881, #14114, #4444, .T. ) ;
#4827=ORIENTED_EDGE ( 'NONE', *, *, #21054, .F. ) ;
#4840=CARTESIAN_POINT ( 'NONE',  ( 0.000000000000000000, 0.000000000000000000, 0.4724409448818898127 ) ) ;
#4848=DIRECTION ( 'NONE',  ( 0.000000000000000000, 0.000000000000000000, 1.000000000000000000 ) ) ;
#4865=EDGE_CURVE ( 'NONE', #22433, #21273, #24422, .T. ) ;
#4866=AXIS2_PLACEMENT_3D ( 'NONE', #24813, #7440, #14243 ) ;
#4868=ADVANCED_FACE ( 'NONE', ( #27225 ), #26512, .F. ) ;
#4877=VERTEX_POINT ( 'NONE', #1104 ) ;
#4890=ORIENTED_EDGE ( 'NONE', *, *, #23604, .F. ) ;
#4891=CIRCLE ( 'NONE', #3444, 0.6881889763779527325 ) ;
#4899=DIRECTION ( 'NONE',  ( -1.000000000000000000, 1.224646799147353454E-16, 0.000000000000000000 ) ) ;
#4924=ORIENTED_EDGE ( 'NONE', *, *, #16663, .T. ) ;
#4954=ORIENTED_EDGE ( 'NONE', *, *, #1628, .F. ) ;
#4958=EDGE_LOOP ( 'NONE', ( #27570, #8645, #7902, #4954 ) ) ;
#4966=DIRECTION ( 'NONE',  ( 0.000000000000000000, 0.000000000000000000, 1.000000000000000000 ) ) ;
#4976=DIRECTION ( 'NONE',  ( -0.7818314824680298036, 0.6234898018587337054, 0.000000000000000000 ) ) ;
#4985=CARTESIAN_POINT ( 'NONE',  ( 0.000000000000000000, 0.000000000000000000, 0.2362204724409449064 ) ) ;
#4986=ORIENTED_EDGE ( 'NONE', *, *, #12754, .F. ) ;
#4999=ADVANCED_FACE ( 'NONE', ( #11896, #18075 ), #24327, .T. ) ;
#5001=CARTESIAN_POINT ( 'NONE',  ( 0.000000000000000000, 0.000000000000000000, 0.2362204724409449064 ) ) ;
#5008=TOROIDAL_SURFACE ( 'NONE', #27072, 0.8031496062992127261, 0.02362204724409448786 ) ;
#5016=ORIENTED_EDGE ( 'NONE', *, *, #7452, .F. ) ;
#5037=DIRECTION ( 'NONE',  ( 1.224646799147353207E-16, 1.000000000000000000, -0.000000000000000000 ) ) ;
#5058=CARTESIAN_POINT ( 'NONE',  ( 0.7214243740402349614, -0.1654689342656808781, 0.2562996996016383422 ) ) ;
#5063=CIRCLE ( 'NONE', #3252, 0.5322834645669292097 ) ;
#5077=DIRECTION ( 'NONE',  ( 0.000000000000000000, 1.000000000000000000, 0.000000000000000000 ) ) ;
#5084=VERTEX_POINT ( 'NONE', #23364 ) ;
#5098=ORIENTED_EDGE ( 'NONE', *, *, #16663, .F. ) ;
#5107=CARTESIAN_POINT ( 'NONE',  ( 0.000000000000000000, 0.000000000000000000, 0.1322834645669291320 ) ) ;
#5108=CARTESIAN_POINT ( 'NONE',  ( -0.5614173959491228771, 0.4467232815856471695, 0.3122824329321748915 ) ) ;
#5114=CARTESIAN_POINT ( 'NONE',  ( 0.2239856983831502169, -0.4635973202131455917, 0.1473214333510785012 ) ) ;
#5127=CARTESIAN_POINT ( 'NONE',  ( 0.0006479495459697544183, 0.5014297259257108896, 0.3080453759639392719 ) ) ;
#5152=DIRECTION ( 'NONE',  ( 0.7818314824680300257, 0.6234898018587330393, -0.000000000000000000 ) ) ;
#5166=ORIENTED_EDGE ( 'NONE', *, *, #2485, .F. ) ;
#5168=FACE_BOUND ( 'NONE', #9635, .T. ) ;
#5174=EDGE_CURVE ( 'NONE', #27602, #1942, #15289, .T. ) ;
#5179=AXIS2_PLACEMENT_3D ( 'NONE', #24097, #13628, #21710 ) ;
#5193=AXIS2_PLACEMENT_3D ( 'NONE', #13555, #2541, #9301 ) ;
#5195=ORIENTED_EDGE ( 'NONE', *, *, #27799, .F. ) ;
#5197=EDGE_CURVE ( 'NONE', #13825, #8723, #4891, .T. ) ;
#5204=ORIENTED_EDGE ( 'NONE', *, *, #17454, .F. ) ;
#5206=CARTESIAN_POINT ( 'NONE',  ( 0.4165721057576322606, 0.3313508221749649763, 0.3401574803149606252 ) ) ;
#5207=EDGE_CURVE ( 'NONE', #24495, #7391, #25132, .T. ) ;
#5224=CARTESIAN_POINT ( 'NONE',  ( 0.2169784220074747749, -0.4520537072447231020, 0.3080453759200848518 ) ) ;
#5226=DIRECTION ( 'NONE',  ( 1.224646799147353207E-16, 1.000000000000000000, -0.000000000000000000 ) ) ;
#5229=CARTESIAN_POINT ( 'NONE',  ( 0.000000000000000000, 0.000000000000000000, 0.000000000000000000 ) ) ;
#5230=EDGE_CURVE ( 'NONE', #11142, #2922, #10315, .T. ) ;
#5233=AXIS2_PLACEMENT_3D ( 'NONE', #25993, #21482, #8208 ) ;
#5244=CARTESIAN_POINT ( 'NONE',  ( 0.2992781133268291316, -0.6197069291944922176, 0.1322834645669291320 ) ) ;
#5258=CARTESIAN_POINT ( 'NONE',  ( -0.2303471512294322787, -0.4798602677570401598, 0.3401574803149606252 ) ) ;
#5264=CARTESIAN_POINT ( 'NONE',  ( 0.000000000000000000, 0.000000000000000000, 0.1322834645669291320 ) ) ;
#5282=CARTESIAN_POINT ( 'NONE',  ( -0.2089723435111595085, -0.4324731448915372645, 0.2194422276631042279 ) ) ;
#5286=DIRECTION ( 'NONE',  ( 0.000000000000000000, 1.000000000000000000, 0.000000000000000000 ) ) ;
#5300=ORIENTED_EDGE ( 'NONE', *, *, #1608, .F. ) ;
#5305=FACE_OUTER_BOUND ( 'NONE', #4175, .T. ) ;
#5329=AXIS2_PLACEMENT_3D ( 'NONE', #24038, #4675, #11179 ) ;
#5337=AXIS2_PLACEMENT_3D ( 'NONE', #20855, #16478, #18575 ) ;
#5370=DIRECTION ( 'NONE',  ( 0.000000000000000000, 0.000000000000000000, 1.000000000000000000 ) ) ;
#5372=CARTESIAN_POINT ( 'NONE',  ( -6.518592411209533944E-17, -0.5322834645669292097, 0.06614173228346456601 ) ) ;
#5373=DIRECTION ( 'NONE',  ( 0.000000000000000000, 1.000000000000000000, 0.000000000000000000 ) ) ;
#5378=ORIENTED_EDGE ( 'NONE', *, *, #23846, .T. ) ;
#5381=ORIENTED_EDGE ( 'NONE', *, *, #15398, .T. ) ;
#5385=CIRCLE ( 'NONE', #8927, 0.5322834645669292097 ) ;
#5392=FACE_OUTER_BOUND ( 'NONE', #16212, .T. ) ;
#5411=CARTESIAN_POINT ( 'NONE',  ( 0.2158067241000556635, -0.4466421405284947688, 0.1734435148016537642 ) ) ;
#5413=CARTESIAN_POINT ( 'NONE',  ( 0.2311492806687369950, -0.4794744477484330636, 0.1322810039474933141 ) ) ;
#5421=CIRCLE ( 'NONE', #21220, 0.02362204724409448786 ) ;
#5436=AXIS2_PLACEMENT_3D ( 'NONE', #12609, #23216, #27733 ) ;
#5444=PRODUCT_CONTEXT ( 'NONE', #9969, 'mechanical' ) ;
#5455=ORIENTED_EDGE ( 'NONE', *, *, #18104, .T. ) ;
#5492=CARTESIAN_POINT ( 'NONE',  ( 0.6709908451338839619, -0.1528902114222553399, 0.3401599409343967761 ) ) ;
#5498=EDGE_LOOP ( 'NONE', ( #16715, #23392, #1461, #22477 ) ) ;
#5509=DIRECTION ( 'NONE',  ( 0.000000000000000000, 0.000000000000000000, 1.000000000000000000 ) ) ;
#5513=CARTESIAN_POINT ( 'NONE',  ( 0.4681308612729632168, -0.1074986424507603650, 0.2529987172375934845 ) ) ;
#5545=CARTESIAN_POINT ( 'NONE',  ( -0.4160174684701755665, 0.3320469875258716397, 0.3401599409343964431 ) ) ;
#5572=EDGE_CURVE ( 'NONE', #24310, #21309, #423, .T. ) ;
#5574=CIRCLE ( 'NONE', #8280, 0.1299232283464567539 ) ;
#5598=CARTESIAN_POINT ( 'NONE',  ( 0.0006679551606482677165, 0.5322830454629158270, 0.3401574803149606252 ) ) ;
#5608=CARTESIAN_POINT ( 'NONE',  ( 0.000000000000000000, 0.000000000000000000, 0.4724409448818898127 ) ) ;
#5622=DIRECTION ( 'NONE',  ( -0.2225209339563147537, -0.9749279121818235083, 0.000000000000000000 ) ) ;
#5630=CARTESIAN_POINT ( 'NONE',  ( 0.000000000000000000, 0.000000000000000000, 0.2362204724409449064 ) ) ;
#5631=ORIENTED_EDGE ( 'NONE', *, *, #14553, .T. ) ;
#5634=ORIENTED_EDGE ( 'NONE', *, *, #18752, .T. ) ;
#5646=CARTESIAN_POINT ( 'NONE',  ( 0.8031496062992127261, 0.000000000000000000, -1.092739370078740131E-17 ) ) ;
#5650=CARTESIAN_POINT ( 'NONE',  ( -0.3882259019046727655, 0.3087756353513817498, 0.2989974301419745517 ) ) ;
#5652=EDGE_LOOP ( 'NONE', ( #9370, #6715, #3313, #11492, #23116, #3279 ) ) ;
#5672=CARTESIAN_POINT ( 'NONE',  ( -0.2988215684304370012, -0.6199272547993012195, 0.3401599409343967761 ) ) ;
#5678=CARTESIAN_POINT ( 'NONE',  ( -0.2315507648392299000, -0.4792806379917101678, 0.3401574803149606252 ) ) ;
#5679=EDGE_CURVE ( 'NONE', #21273, #23783, #24290, .T. ) ;
#5702=VERTEX_POINT ( 'NONE', #15054 ) ;
#5717=VERTEX_POINT ( 'NONE', #23668 ) ;
#5732=ORIENTED_EDGE ( 'NONE', *, *, #4509, .T. ) ;
#5734=DIRECTION ( 'NONE',  ( 1.000000000000000000, 0.000000000000000000, 0.000000000000000000 ) ) ;
#5742=CARTESIAN_POINT ( 'NONE',  ( 0.2146455952141596568, -0.4472013107316724079, 0.1734435147974487113 ) ) ;
#5766=LINE ( 'NONE', #6191, #9622 ) ;
#5825=ORIENTED_EDGE ( 'NONE', *, *, #14340, .F. ) ;
#5826=CARTESIAN_POINT ( 'NONE',  ( -0.2992781133269515892, -0.6197069291944330427, 0.1322834645669291320 ) ) ;
#5843=ADVANCED_FACE ( 'NONE', ( #27830, #17088 ), #14986, .T. ) ;
#5870=ORIENTED_EDGE ( 'NONE', *, *, #1565, .T. ) ;
#5888=VERTEX_POINT ( 'NONE', #6836 ) ;
#5898=CARTESIAN_POINT ( 'NONE',  ( 0.000000000000000000, 0.8267716535433071723, 0.2362204724409449064 ) ) ;
#5914=EDGE_CURVE ( 'NONE', #1942, #16391, #22730, .T. ) ;
#5920=EDGE_CURVE ( 'NONE', #23881, #15279, #6868, .T. ) ;
#5935=EDGE_CURVE ( 'NONE', #9678, #24096, #9875, .T. ) ;
#5945=CARTESIAN_POINT ( 'NONE',  ( -0.0006679551606482677165, 0.5322830454629158270, 0.1322834645669291320 ) ) ;
#5948=AXIS2_PLACEMENT_3D ( 'NONE', #14923, #25348, #18555 ) ;
#5951=VERTEX_POINT ( 'NONE', #7549 ) ;
#5955=CARTESIAN_POINT ( 'NONE',  ( -0.3218523081051654078, -0.6665164569871881994, 0.2562996995972176006 ) ) ;
#5958=CARTESIAN_POINT ( 'NONE',  ( -0.2983664441502653641, -0.6201464311010354002, 0.3401599409343967761 ) ) ;
#5967=EDGE_LOOP ( 'NONE', ( #27752, #644 ) ) ;
#5989=CARTESIAN_POINT ( 'NONE',  ( 0.000000000000000000, 0.000000000000000000, 0.3401574803149606252 ) ) ;
#5998=CARTESIAN_POINT ( 'NONE',  ( 0.2181459867445876555, -0.4514914376998327428, 0.3080453759178627404 ) ) ;
#6014=AXIS2_PLACEMENT_3D ( 'NONE', #17406, #17802, #15319 ) ;
#6017=CARTESIAN_POINT ( 'NONE',  ( -1.012503259137575512E-16, -0.8267716535433071723, 0.4488188976377953110 ) ) ;
#6032=DIRECTION ( 'NONE',  ( 0.000000000000000000, -1.000000000000000000, 0.000000000000000000 ) ) ;
#6050=CARTESIAN_POINT ( 'NONE',  ( 0.000000000000000000, 0.000000000000000000, 0.3401574803149606252 ) ) ;
#6076=CARTESIAN_POINT ( 'NONE',  ( -0.2078289949484353749, -0.4330237525397954146, 0.2529987172201150769 ) ) ;
#6093=DIRECTION ( 'NONE',  ( 0.000000000000000000, -1.000000000000000000, 0.000000000000000000 ) ) ;
#6109=CARTESIAN_POINT ( 'NONE',  ( -0.0002221395201540944610, 0.5322834645669292097, 0.3401599409343964431 ) ) ;
#6110=CARTESIAN_POINT ( 'NONE',  ( -0.2158067241058057306, -0.4466421405404321088, 0.2989974301043377136 ) ) ;
#6129=ORIENTED_EDGE ( 'NONE', *, *, #15873, .T. ) ;
#6139=CARTESIAN_POINT ( 'NONE',  ( 0.000000000000000000, 0.000000000000000000, 0.02362204724409448786 ) ) ;
#6146=CARTESIAN_POINT ( 'NONE',  ( 0.2158067241018476468, -0.4466421405321954752, 0.2989974300877151769 ) ) ;
#6168=ORIENTED_EDGE ( 'NONE', *, *, #1068, .T. ) ;
#6188=CARTESIAN_POINT ( 'NONE',  ( -0.6711032387266713251, -0.1523958994812759926, 0.3401574803149606252 ) ) ;
#6191=CARTESIAN_POINT ( 'NONE',  ( 0.000000000000000000, 0.5322834645669292097, 0.06614173228346456601 ) ) ;
#6198=AXIS2_PLACEMENT_3D ( 'NONE', #21910, #15561, #23760 ) ;
#6199=ORIENTED_EDGE ( 'NONE', *, *, #25903, .T. ) ;
#6216=DIRECTION ( 'NONE',  ( 0.000000000000000000, 0.000000000000000000, 1.000000000000000000 ) ) ;
#6235=CARTESIAN_POINT ( 'NONE',  ( 0.0007882571242852967879, 0.7401570605731624397, 0.2161412452768986248 ) ) ;
#6248=DIRECTION ( 'NONE',  ( 0.000000000000000000, -1.000000000000000000, 0.000000000000000000 ) ) ;
#6272=AXIS2_PLACEMENT_3D ( 'NONE', #11216, #23948, #9220 ) ;
#6286=B_SPLINE_CURVE_WITH_KNOTS ( 'NONE', 3,
 ( #819, #7171, #26950, #15793, #9408, #24260 ),
 .UNSPECIFIED., .F., .F.,
 ( 4, 2, 4 ),
 ( 0.3864984308775630262, 0.3881911340211379735, 0.3898838371647110335 ),
 .UNSPECIFIED. ) ;
#6319=CIRCLE ( 'NONE', #27538, 0.4173228346456693272 ) ;
#6321=CARTESIAN_POINT ( 'NONE',  ( 0.5375739373539409893, 0.4296723508511047229, 0.1322834645669291320 ) ) ;
#6328=CIRCLE ( 'NONE', #13981, 0.1299232283464566984 ) ;
#6332=VERTEX_POINT ( 'NONE', #18146 ) ;
#6339=ORIENTED_EDGE ( 'NONE', *, *, #22252, .T. ) ;
#6345=ORIENTED_EDGE ( 'NONE', *, *, #6623, .T. ) ;
#6372=ORIENTED_EDGE ( 'NONE', *, *, #5207, .F. ) ;
#6374=DIRECTION ( 'NONE',  ( 0.000000000000000000, 0.000000000000000000, 1.000000000000000000 ) ) ;
#6377=EDGE_CURVE ( 'NONE', #8989, #11425, #16909, .T. ) ;
#6422=CARTESIAN_POINT ( 'NONE',  ( 0.000000000000000000, 0.000000000000000000, 0.3401574803149606252 ) ) ;
#6446=CARTESIAN_POINT ( 'NONE',  ( 0.4165721057576322606, 0.3313508221749649763, 0.1322834645669291320 ) ) ;
#6453=AXIS2_PLACEMENT_3D ( 'NONE', #26750, #24486, #18401 ) ;
#6454=VERTEX_POINT ( 'NONE', #23277 ) ;
#6479=AXIS2_PLACEMENT_3D ( 'NONE', #739, #15989, #20363 ) ;
#6485=TOROIDAL_SURFACE ( 'NONE', #21367, 0.6102362204724409711, 0.1299212598425196763 ) ;
#6492=CARTESIAN_POINT ( 'NONE',  ( -0.0006362927944362226432, 0.4836123550485326716, 0.2715646632801987925 ) ) ;
#6494=CARTESIAN_POINT ( 'NONE',  ( -0.2647715730835492609, -0.5498038367121063086, 0.2362204724409449064 ) ) ;
#6501=FACE_OUTER_BOUND ( 'NONE', #996, .T. ) ;
#6509=CARTESIAN_POINT ( 'NONE',  ( 0.3785000865565943395, 0.3010298976875371291, 0.2715646632839407437 ) ) ;
#6524=DIRECTION ( 'NONE',  ( 0.4338837391175580094, -0.9009688679024192570, 0.000000000000000000 ) ) ;
#6530=ORIENTED_EDGE ( 'NONE', *, *, #2877, .T. ) ;
#6533=AXIS2_PLACEMENT_3D ( 'NONE', #43, #8605, #24534 ) ;
#6537=DIRECTION ( 'NONE',  ( 0.000000000000000000, 1.000000000000000000, 0.000000000000000000 ) ) ;
#6538=EDGE_CURVE ( 'NONE', #5084, #11259, #25716, .T. ) ;
#6542=VERTEX_POINT ( 'NONE', #4464 ) ;
#6570=CARTESIAN_POINT ( 'NONE',  ( -0.6707652279343347956, -0.1538768215240151616, 0.3401574803149606252 ) ) ;
#6572=AXIS2_PLACEMENT_3D ( 'NONE', #9486, #7674, #14179 ) ;
#6577=CARTESIAN_POINT ( 'NONE',  ( 0.5190368482393039606, -0.1180105360553401483, 0.1322818204150990051 ) ) ;
#6584=CARTESIAN_POINT ( 'NONE',  ( -0.2169784220102915218, -0.4520537072505400045, 0.3080453759295606053 ) ) ;
#6587=VECTOR ( 'NONE', #22593, 39.37007874015748143 ) ;
#6603=VERTEX_POINT ( 'NONE', #9988 ) ;
#6620=ORIENTED_EDGE ( 'NONE', *, *, #16004, .T. ) ;
#6623=EDGE_CURVE ( 'NONE', #22088, #16756, #3566, .T. ) ;
#6631=EDGE_CURVE ( 'NONE', #7391, #27673, #25021, .T. ) ;
#6632=FACE_OUTER_BOUND ( 'NONE', #20173, .T. ) ;
#6638=CARTESIAN_POINT ( 'NONE',  ( -0.5189874374926378708, -0.1182276436463389618, 0.1322810039474935084 ) ) ;
#6650=CARTESIAN_POINT ( 'NONE',  ( -0.3785000865568526884, 0.3010298976877424648, 0.2008762815967665150 ) ) ;
#6653=EDGE_LOOP ( 'NONE', ( #3461, #12252 ) ) ;
#6658=CARTESIAN_POINT ( 'NONE',  ( -0.0007595033562148819414, 0.6881885572739390167, 0.3401574803149606252 ) ) ;
#6680=EDGE_CURVE ( 'NONE', #17014, #11142, #12214, .T. ) ;
#6689=CARTESIAN_POINT ( 'NONE',  ( -0.2078289949484350141, -0.4330237525397957477, 0.2362204724409447676 ) ) ;
#6704=CARTESIAN_POINT ( 'NONE',  ( 5.827097576719993621E-17, 0.6881889763779529545, 0.3401599409343964431 ) ) ;
#6705=FACE_OUTER_BOUND ( 'NONE', #16059, .T. ) ;
#6712=DIRECTION ( 'NONE',  ( 0.000000000000000000, 0.000000000000000000, 1.000000000000000000 ) ) ;
#6715=ORIENTED_EDGE ( 'NONE', *, *, #12974, .F. ) ;
#6729=DIRECTION ( 'NONE',  ( 1.000000000000000000, 0.000000000000000000, 0.000000000000000000 ) ) ;
#6730=ORIENTED_EDGE ( 'NONE', *, *, #20658, .T. ) ;
#6735=ORIENTED_EDGE ( 'NONE', *, *, #9476, .T. ) ;
#6754=ORIENTED_EDGE ( 'NONE', *, *, #21479, .T. ) ;
#6775=CARTESIAN_POINT ( 'NONE',  ( 0.000000000000000000, 0.6881889763779527325, 0.06614173228346456601 ) ) ;
#6788=B_SPLINE_CURVE_WITH_KNOTS ( 'NONE', 3,
 ( #21972, #6862, #23956, #24088 ),
 .UNSPECIFIED., .F., .F.,
 ( 4, 4 ),
 ( 0.4045103800602309896, 0.4064350009536160102 ),
 .UNSPECIFIED. ) ;
#6808=CARTESIAN_POINT ( 'NONE',  ( -0.5190862322091315262, -0.1177929122753175184, 0.3401574803149606252 ) ) ;
#6826=CARTESIAN_POINT ( 'NONE',  ( 0.000000000000000000, 0.000000000000000000, 0.2362204724409449064 ) ) ;
#6828=CARTESIAN_POINT ( 'NONE',  ( -0.2078289949484354027, -0.4330237525397954146, 0.2194422276617741807 ) ) ;
#6836=CARTESIAN_POINT ( 'NONE',  ( 0.2647715730835492609, -0.5498038367121063086, 0.3661437007874016047 ) ) ;
#6837=DIRECTION ( 'NONE',  ( 0.000000000000000000, 0.000000000000000000, 1.000000000000000000 ) ) ;
#6859=CARTESIAN_POINT ( 'NONE',  ( -0.2092582568878602056, -0.4359957531173518364, 0.2715646632357672785 ) ) ;
#6862=CARTESIAN_POINT ( 'NONE',  ( 0.0005057506112066535546, 0.6881888373222776467, 0.1322818203437346463 ) ) ;
#6868=B_SPLINE_CURVE_WITH_KNOTS ( 'NONE', 3,
 ( #2444, #9075, #21810, #7842, #3569, #20550, #11641, #16447 ),
 .UNSPECIFIED., .F., .F.,
 ( 4, 2, 2, 4 ),
 ( 0.5000000000000000000, 0.7499999999999996669, 0.8749999999999997780, 1.000000000000000000 ),
 .UNSPECIFIED. ) ;
#6879=CARTESIAN_POINT ( 'NONE',  ( 0.5510854067045450888, 0.4384931681290698546, 0.1443310008641096598 ) ) ;
#6886=EDGE_LOOP ( 'NONE', ( #17915, #414, #18388, #8067, #26558 ) ) ;
#6889=CARTESIAN_POINT ( 'NONE',  ( 0.000000000000000000, 0.000000000000000000, 0.3401574803149606252 ) ) ;
#6890=ORIENTED_EDGE ( 'NONE', *, *, #5230, .T. ) ;
#6900=ADVANCED_FACE ( 'NONE', ( #14565 ), #26601, .F. ) ;
#6911=CARTESIAN_POINT ( 'NONE',  ( 0.0006620872580302083164, 0.5229309616567520136, 0.1392975274215518533 ) ) ;
#6917=DIRECTION ( 'NONE',  ( 1.000000000000000000, 0.000000000000000000, 0.000000000000000000 ) ) ;
#6918=AXIS2_PLACEMENT_3D ( 'NONE', #178, #4517, #6917 ) ;
#6936=DIRECTION ( 'NONE',  ( 0.000000000000000000, 0.000000000000000000, -1.000000000000000000 ) ) ;
#6940=FACE_OUTER_BOUND ( 'NONE', #523, .T. ) ;
#6959=FACE_OUTER_BOUND ( 'NONE', #1577, .T. ) ;
#6969=CARTESIAN_POINT ( 'NONE',  ( 0.000000000000000000, 0.000000000000000000, 0.1322834645669291320 ) ) ;
#6972=EDGE_CURVE ( 'NONE', #25110, #22690, #13514, .T. ) ;
#6977=CARTESIAN_POINT ( 'NONE',  ( -0.5385210225480960844, 0.4284847435812472183, 0.1322834645669291320 ) ) ;
#6979=CARTESIAN_POINT ( 'NONE',  ( 0.2305483297598421022, -0.4797636960996590760, 0.3401591244667909186 ) ) ;
#6982=FACE_BOUND ( 'NONE', #1206, .T. ) ;
#7009=CARTESIAN_POINT ( 'NONE',  ( 0.4021324607176451904, 0.3215300179777050293, 0.3251195115651615564 ) ) ;
#7010=DIRECTION ( 'NONE',  ( 0.000000000000000000, 0.000000000000000000, 1.000000000000000000 ) ) ;
#7020=CARTESIAN_POINT ( 'NONE',  ( 0.4837521785364486404, -0.1097523286759638783, 0.1734435147541967814 ) ) ;
#7023=CIRCLE ( 'NONE', #8809, 0.3937007874015748254 ) ;
#7027=DIRECTION ( 'NONE',  ( 0.000000000000000000, 0.000000000000000000, 1.000000000000000000 ) ) ;
#7029=CIRCLE ( 'NONE', #21936, 0.5322834645669292097 ) ;
#7081=CARTESIAN_POINT ( 'NONE',  ( -0.4681308612729632723, -0.1074986424507606286, 0.2194422276514244319 ) ) ;
#7117=CARTESIAN_POINT ( 'NONE',  ( 0.000000000000000000, 0.000000000000000000, 0.2362204724409449064 ) ) ;
#7141=ORIENTED_EDGE ( 'NONE', *, *, #1718, .F. ) ;
#7142=CARTESIAN_POINT ( 'NONE',  ( -0.4157391792961063204, 0.3323952789219086768, 0.1322834645669291320 ) ) ;
#7151=CARTESIAN_POINT ( 'NONE',  ( 0.000000000000000000, 0.000000000000000000, 0.3401574803149606252 ) ) ;
#7159=ORIENTED_EDGE ( 'NONE', *, *, #17574, .T. ) ;
#7168=DIRECTION ( 'NONE',  ( 1.000000000000000000, 0.000000000000000000, 0.000000000000000000 ) ) ;
#7171=CARTESIAN_POINT ( 'NONE',  ( -0.2305483297598421022, -0.4797636960996590760, 0.1322818204150988386 ) ) ;
#7174=DIRECTION ( 'NONE',  ( 0.000000000000000000, 0.000000000000000000, 1.000000000000000000 ) ) ;
#7185=ORIENTED_EDGE ( 'NONE', *, *, #5197, .T. ) ;
#7187=CARTESIAN_POINT ( 'NONE',  ( 0.6993003464534486291, -0.1604063846362702717, 0.1601585119470639862 ) ) ;
#7188=B_SPLINE_CURVE_WITH_KNOTS ( 'NONE', 3,
 ( #9928, #3708, #21090, #20949, #27743, #7823, #25612, #16431, #21379, #25048 ),
 .UNSPECIFIED., .F., .F.,
 ( 4, 2, 2, 2, 4 ),
 ( 0.000000000000000000, 0.2500000000000000000, 0.5000000000000000000, 0.7500000000000000000, 1.000000000000000000 ),
 .UNSPECIFIED. ) ;
#7198=CARTESIAN_POINT ( 'NONE',  ( 0.000000000000000000, 0.000000000000000000, 0.4488188976377953110 ) ) ;
#7204=CARTESIAN_POINT ( 'NONE',  ( 0.6711032387266713251, -0.1523958994812761869, 0.3401574803149606252 ) ) ;
#7205=CARTESIAN_POINT ( 'NONE',  ( 0.000000000000000000, 0.6102362204724409711, -1.156053543307086666E-17 ) ) ;
#7225=FACE_OUTER_BOUND ( 'NONE', #28, .T. ) ;
#7229=EDGE_CURVE ( 'NONE', #16925, #26228, #10851, .T. ) ;
#7243=( NAMED_UNIT ( * ) PLANE_ANGLE_UNIT ( ) SI_UNIT ( $, .RADIAN. ) ) ;
#7245=CARTESIAN_POINT ( 'NONE',  ( -1.012503259137575512E-16, -0.8267716535433071723, 0.2362204724409449064 ) ) ;
#7274=CARTESIAN_POINT ( 'NONE',  ( 0.4684132450478840082, -0.1062614382955253955, 0.2529987172365008030 ) ) ;
#7292=ORIENTED_EDGE ( 'NONE', *, *, #18293, .F. ) ;
#7299=CARTESIAN_POINT ( 'NONE',  ( -0.3937007874015748254, 4.966087413865251393E-17, 0.4488188976377953110 ) ) ;
#7318=EDGE_LOOP ( 'NONE', ( #20741, #23290, #16224, #11357, #2992 ) ) ;
#7325=ORIENTED_EDGE ( 'NONE', *, *, #16824, .F. ) ;
#7346=FACE_BOUND ( 'NONE', #6653, .T. ) ;
#7359=CARTESIAN_POINT ( 'NONE',  ( -0.2992781133269515892, -0.6197069291944330427, 0.3401574803149606252 ) ) ;
#7366=EDGE_CURVE ( 'NONE', #21655, #6603, #12661, .T. ) ;
#7377=DIRECTION ( 'NONE',  ( 0.000000000000000000, 0.000000000000000000, 1.000000000000000000 ) ) ;
#7381=CARTESIAN_POINT ( 'NONE',  ( 0.2990496115119744003, -0.6198172806990825956, 0.3401591245381555551 ) ) ;
#7388=EDGE_CURVE ( 'NONE', #15279, #15981, #489, .T. ) ;
#7391=VERTEX_POINT ( 'NONE', #2900 ) ;
#7397=ADVANCED_FACE ( 'NONE', ( #5168, #20150 ), #11813, .T. ) ;
#7408=ORIENTED_EDGE ( 'NONE', *, *, #24538, .T. ) ;
#7412=CARTESIAN_POINT ( 'NONE',  ( 0.5744851493189444547, 0.4591414886171028553, 0.2763636194376414279 ) ) ;
#7440=DIRECTION ( 'NONE',  ( 0.000000000000000000, 0.000000000000000000, 1.000000000000000000 ) ) ;
#7442=CIRCLE ( 'NONE', #6572, 0.1299232283464566984 ) ;
#7445=CARTESIAN_POINT ( 'NONE',  ( 0.000000000000000000, 0.8267716535433071723, 0.4488188976377953110 ) ) ;
#7448=DIRECTION ( 'NONE',  ( 0.000000000000000000, 0.000000000000000000, 1.000000000000000000 ) ) ;
#7451=TOROIDAL_SURFACE ( 'NONE', #2058, 0.6102362204724409711, 0.1299212598425196763 ) ;
#7452=EDGE_CURVE ( 'NONE', #18836, #19875, #27112, .T. ) ;
#7453=ORIENTED_EDGE ( 'NONE', *, *, #5230, .F. ) ;
#7456=DIRECTION ( 'NONE',  ( 1.000000000000000000, 0.000000000000000000, 0.000000000000000000 ) ) ;
#7483=CARTESIAN_POINT ( 'NONE',  ( 0.000000000000000000, 0.000000000000000000, 0.4724409448818898127 ) ) ;
#7485=AXIS2_PLACEMENT_3D ( 'NONE', #10802, #4309, #25782 ) ;
#7505=B_SPLINE_CURVE_WITH_KNOTS ( 'NONE', 3,
 ( #548, #6911, #23736, #20030, #11139, #21612, #19757, #15534 ),
 .UNSPECIFIED., .F., .F.,
 ( 4, 2, 2, 4 ),
 ( 0.000000000000000000, 0.1249999999999998335, 0.2499999999999997780, 0.5000000000000000000 ),
 .UNSPECIFIED. ) ;
#7508=ADVANCED_FACE ( 'NONE', ( #26936, #11959 ), #7728, .T. ) ;
#7527=CARTESIAN_POINT ( 'NONE',  ( -0.4157391792961063204, 0.3323952789219086768, 0.1322834645669291320 ) ) ;
#7531=ORIENTED_EDGE ( 'NONE', *, *, #967, .T. ) ;
#7546=VERTEX_POINT ( 'NONE', #7575 ) ;
#7549=CARTESIAN_POINT ( 'NONE',  ( 0.000000000000000000, 0.6881889763779527325, 0.1322810039474933141 ) ) ;
#7558=AXIS2_PLACEMENT_3D ( 'NONE', #8425, #17316, #19581 ) ;
#7575=CARTESIAN_POINT ( 'NONE',  ( 0.6707652279343464530, -0.1538768215239712522, 0.1322834645669291320 ) ) ;
#7581=TOROIDAL_SURFACE ( 'NONE', #25635, 0.8031496062992127261, 0.02362204724409448786 ) ;
#7600=CARTESIAN_POINT ( 'NONE',  ( 0.5949363243629232079, -0.1357903337134992172, 0.2362204724409449064 ) ) ;
#7605=EDGE_LOOP ( 'NONE', ( #1814, #24887, #23706, #4426 ) ) ;
#7609=DIRECTION ( 'NONE',  ( 0.9749279121818235083, -0.2225209339563150035, 0.000000000000000000 ) ) ;
#7634=LINE ( 'NONE', #5372, #27256 ) ;
#7637=DIRECTION ( 'NONE',  ( 0.000000000000000000, 0.000000000000000000, 1.000000000000000000 ) ) ;
#7645=CARTESIAN_POINT ( 'NONE',  ( -0.3218523081044682987, -0.6665164569857464638, 0.2161412452743130541 ) ) ;
#7674=DIRECTION ( 'NONE',  ( 0.000000000000000000, -1.000000000000000000, 0.000000000000000000 ) ) ;
#7697=EDGE_CURVE ( 'NONE', #10270, #9314, #14969, .T. ) ;
#7710=CARTESIAN_POINT ( 'NONE',  ( 0.5781866216489107702, 0.4620966632771911220, 0.2161412452773199544 ) ) ;
#7726=EDGE_LOOP ( 'NONE', ( #12124, #7531, #19942, #14707 ) ) ;
#7728=SPHERICAL_SURFACE ( 'NONE', #27559, 0.1299232283464566984 ) ;
#7764=ORIENTED_EDGE ( 'NONE', *, *, #2229, .T. ) ;
#7771=TOROIDAL_SURFACE ( 'NONE', #23573, 0.6102362204724409711, 0.1299212598425196763 ) ;
#7785=VECTOR ( 'NONE', #16974, 39.37007874015748143 ) ;
#7823=CARTESIAN_POINT ( 'NONE',  ( -0.0007882571242873708667, 0.7401570605738059250, 0.2562996996008273243 ) ) ;
#7837=CARTESIAN_POINT ( 'NONE',  ( -0.4837521785345547665, -0.1097523286755377608, 0.1734435147577276792 ) ) ;
#7842=CARTESIAN_POINT ( 'NONE',  ( -0.0006443779181934992202, 0.4960456921228240112, 0.1734435147396095056 ) ) ;
#7856=AXIS2_PLACEMENT_3D ( 'NONE', #7205, #13697, #22180 ) ;
#7862=CARTESIAN_POINT ( 'NONE',  ( -0.2089723435111590921, -0.4324731448915377641, 0.2362204724409450174 ) ) ;
#7866=B_SPLINE_CURVE_WITH_KNOTS ( 'NONE', 3,
 ( #22566, #11543, #11682, #13809, #1243, #22425, #962, #3191, #11824, #8162 ),
 .UNSPECIFIED., .F., .F.,
 ( 4, 2, 2, 2, 4 ),
 ( 0.000000000000000000, 0.2499999999999998890, 0.4999999999999997780, 0.7499999999999996669, 1.000000000000000000 ),
 .UNSPECIFIED. ) ;
#7868=DIRECTION ( 'NONE',  ( 0.000000000000000000, 0.000000000000000000, -1.000000000000000000 ) ) ;
#7873=CIRCLE ( 'NONE', #1102, 0.5322834645669292097 ) ;
#7884=DIRECTION ( 'NONE',  ( 0.000000000000000000, 0.000000000000000000, 1.000000000000000000 ) ) ;
#7887=ORIENTED_EDGE ( 'NONE', *, *, #267, .T. ) ;
#7891=EDGE_CURVE ( 'NONE', #9309, #17480, #14035, .T. ) ;
#7896=ORIENTED_EDGE ( 'NONE', *, *, #25971, .F. ) ;
#7900=ORIENTED_EDGE ( 'NONE', *, *, #3968, .F. ) ;
#7902=ORIENTED_EDGE ( 'NONE', *, *, #21479, .F. ) ;
#7906=FACE_OUTER_BOUND ( 'NONE', #2524, .T. ) ;
#7923=DIRECTION ( 'NONE',  ( 1.000000000000000000, 0.000000000000000000, 0.000000000000000000 ) ) ;
#7930=EDGE_LOOP ( 'NONE', ( #7325, #19866, #12446, #10698, #12578, #11251, #20816, #24832, #10076, #19881, #7900 ) ) ;
#7936=CARTESIAN_POINT ( 'NONE',  ( -0.2239856983880364194, -0.4635973202232746559, 0.3251195115423166637 ) ) ;
#7943=DIRECTION ( 'NONE',  ( 0.000000000000000000, 1.000000000000000000, 0.000000000000000000 ) ) ;
#7952=CARTESIAN_POINT ( 'NONE',  ( -0.4165721057576322606, 0.3313508221749649763, 0.3401574803149606252 ) ) ;
#7956=CARTESIAN_POINT ( 'NONE',  ( 0.2089723435111816296, -0.4324731448915269394, 0.2194422276813851325 ) ) ;
#7961=CARTESIAN_POINT ( 'NONE',  ( 0.4771018889076559244, 0.3804760601893846794, 0.2362204724409449064 ) ) ;
#7962=DIRECTION ( 'NONE',  ( 0.000000000000000000, 0.000000000000000000, 1.000000000000000000 ) ) ;
#7964=DIRECTION ( 'NONE',  ( 0.000000000000000000, 0.000000000000000000, 1.000000000000000000 ) ) ;
#7972=EDGE_LOOP ( 'NONE', ( #26711, #3602, #23155, #23238 ) ) ;
#7973=CARTESIAN_POINT ( 'NONE',  ( 0.2979095355689177493, -0.6203660015065670663, 0.3401574803149606252 ) ) ;
#8020=DIRECTION ( 'NONE',  ( 0.000000000000000000, 0.000000000000000000, 1.000000000000000000 ) ) ;
#8026=DIRECTION ( 'NONE',  ( 0.000000000000000000, 0.000000000000000000, -1.000000000000000000 ) ) ;
#8039=DIRECTION ( 'NONE',  ( 0.000000000000000000, 1.000000000000000000, 0.000000000000000000 ) ) ;
#8045=DIRECTION ( 'NONE',  ( -0.9749279121818236193, -0.2225209339563142819, 0.000000000000000000 ) ) ;
#8051=CARTESIAN_POINT ( 'NONE',  ( 0.2647715730835492609, -0.5498038367121063086, 0.2362204724409449064 ) ) ;
#8067=ORIENTED_EDGE ( 'NONE', *, *, #23140, .T. ) ;
#8072=CARTESIAN_POINT ( 'NONE',  ( 0.4173228346456693272, 0.000000000000000000, -5.463696850393700654E-18 ) ) ;
#8074=CARTESIAN_POINT ( 'NONE',  ( -0.2981382804007346454, -0.6202561546315846774, 0.3401591245381551110 ) ) ;
#8094=CIRCLE ( 'NONE', #9874, 0.8267716535433071723 ) ;
#8139=ORIENTED_EDGE ( 'NONE', *, *, #15121, .T. ) ;
#8162=CARTESIAN_POINT ( 'NONE',  ( -0.6707652279343347956, -0.1538768215240151616, 0.3401574803149606252 ) ) ;
#8166=CARTESIAN_POINT ( 'NONE',  ( -0.4165721057576322606, 0.3313508221749649763, 0.3401574803149606252 ) ) ;
#8188=EDGE_CURVE ( 'NONE', #27673, #5084, #27682, .T. ) ;
#8195=AXIS2_PLACEMENT_3D ( 'NONE', #16866, #2016, #13030 ) ;
#8202=ORIENTED_EDGE ( 'NONE', *, *, #1809, .F. ) ;
#8208=DIRECTION ( 'NONE',  ( 1.000000000000000000, 0.000000000000000000, 0.000000000000000000 ) ) ;
#8233=TOROIDAL_SURFACE ( 'NONE', #18587, 0.6102362204724409711, 0.1299212598425196763 ) ;
#8243=EDGE_CURVE ( 'NONE', #11425, #4356, #23553, .T. ) ;
#8251=DIRECTION ( 'NONE',  ( 0.000000000000000000, 0.000000000000000000, 1.000000000000000000 ) ) ;
#8277=ORIENTED_EDGE ( 'NONE', *, *, #2268, .F. ) ;
#8280=AXIS2_PLACEMENT_3D ( 'NONE', #23766, #6524, #21641 ) ;
#8321=CARTESIAN_POINT ( 'NONE',  ( 0.000000000000000000, 0.3937007874015748254, 0.4488188976377953110 ) ) ;
#8353=CARTESIAN_POINT ( 'NONE',  ( -0.4029514798614846072, 0.3205030004507355978, 0.1473214333197954140 ) ) ;
#8356=AXIS2_PLACEMENT_3D ( 'NONE', #136, #10829, #25534 ) ;
#8359=CARTESIAN_POINT ( 'NONE',  ( 0.5377323685532543474, 0.4294741335735771659, 0.3401591245381551110 ) ) ;
#8361=LINE ( 'NONE', #19366, #7785 ) ;
#8394=CIRCLE ( 'NONE', #22823, 0.5322834645669292097 ) ;
#8397=EDGE_LOOP ( 'NONE', ( #21774, #14914, #4827, #3222, #26384, #25952 ) ) ;
#8401=EDGE_CURVE ( 'NONE', #17480, #22690, #12236, .T. ) ;
#8407=FACE_OUTER_BOUND ( 'NONE', #7318, .T. ) ;
#8419=DIRECTION ( 'NONE',  ( 1.000000000000000000, 0.000000000000000000, 0.000000000000000000 ) ) ;
#8425=CARTESIAN_POINT ( 'NONE',  ( 0.000000000000000000, 0.000000000000000000, 0.4724409448818898127 ) ) ;
#8480=CARTESIAN_POINT ( 'NONE',  ( 0.0007856387884314597293, 0.7354206117110280161, 0.2763636194372742216 ) ) ;
#8495=CARTESIAN_POINT ( 'NONE',  ( 0.6709908451338799651, -0.1528902114222700781, 0.1322810039474933141 ) ) ;
#8497=CARTESIAN_POINT ( 'NONE',  ( -0.2078289949484350141, -0.4330237525397957477, 0.2362204724409447676 ) ) ;
#8517=CARTESIAN_POINT ( 'NONE',  ( 0.6711032387266614441, -0.1523958994813204848, 0.1322834645669291320 ) ) ;
#8546=CARTESIAN_POINT ( 'NONE',  ( -8.427884271297532088E-17, -0.6881889763779527325, 0.3401574803149606252 ) ) ;
#8549=EDGE_LOOP ( 'NONE', ( #8666, #1300, #15830, #1491, #6372, #15652 ) ) ;
#8566=B_SPLINE_CURVE_WITH_KNOTS ( 'NONE', 3,
 ( #20657, #16286, #5545, #16417, #18231, #7952 ),
 .UNSPECIFIED., .F., .F.,
 ( 4, 2, 4 ),
 ( 1.162880698919837918, 1.164573402063411978, 1.166266105206986037 ),
 .UNSPECIFIED. ) ;
#8600=CARTESIAN_POINT ( 'NONE',  ( 0.000000000000000000, 0.000000000000000000, 0.02362204724409448786 ) ) ;
#8605=DIRECTION ( 'NONE',  ( 0.000000000000000000, 0.000000000000000000, 1.000000000000000000 ) ) ;
#8619=ADVANCED_FACE ( 'NONE', ( #2431 ), #7771, .F. ) ;
#8627=FACE_OUTER_BOUND ( 'NONE', #10739, .T. ) ;
#8645=ORIENTED_EDGE ( 'NONE', *, *, #4507, .F. ) ;
#8653=CARTESIAN_POINT ( 'NONE',  ( 0.5949363243629232079, -0.1357903337134992172, 0.2362204724409449064 ) ) ;
#8666=ORIENTED_EDGE ( 'NONE', *, *, #22284, .F. ) ;
#8671=CARTESIAN_POINT ( 'NONE',  ( -0.5604501195268866143, 0.4479362078580881312, 0.3122824329294420775 ) ) ;
#8681=PRODUCT_DEFINITION_SHAPE ( 'NONE', 'NONE',  #17410 ) ;
#8685=AXIS2_PLACEMENT_3D ( 'NONE', #24793, #9960, #20569 ) ;
#8693=DIRECTION ( 'NONE',  ( 0.000000000000000000, 1.000000000000000000, 0.000000000000000000 ) ) ;
#8694=EDGE_CURVE ( 'NONE', #20821, #5717, #23639, .T. ) ;
#8696=DIRECTION ( 'NONE',  ( 0.000000000000000000, 0.000000000000000000, 1.000000000000000000 ) ) ;
#8723=VERTEX_POINT ( 'NONE', #25013 ) ;
#8745=CARTESIAN_POINT ( 'NONE',  ( -0.5187889641967551313, -0.1190953285357212593, 0.1322834645669291320 ) ) ;
#8760=CARTESIAN_POINT ( 'NONE',  ( 5.827097576719993621E-17, 0.6881889763779529545, 0.3401599409343964431 ) ) ;
#8780=CIRCLE ( 'NONE', #257, 0.6881889763779527325 ) ;
#8795=DIRECTION ( 'NONE',  ( 0.000000000000000000, 0.000000000000000000, 1.000000000000000000 ) ) ;
#8807=DIRECTION ( 'NONE',  ( 0.000000000000000000, 1.000000000000000000, 0.000000000000000000 ) ) ;
#8808=CARTESIAN_POINT ( 'NONE',  ( -0.5781866216478808163, 0.4620966632763692794, 0.2161412452687943575 ) ) ;
#8809=AXIS2_PLACEMENT_3D ( 'NONE', #6139, #7964, #20808 ) ;
#8818=FACE_OUTER_BOUND ( 'NONE', #17481, .T. ) ;
#8837=CIRCLE ( 'NONE', #7485, 0.02362204724409448092 ) ;
#8840=CARTESIAN_POINT ( 'NONE',  ( 0.4084310843292833226, 0.3265597623332965882, 0.3331434174623317257 ) ) ;
#8844=ORIENTED_EDGE ( 'NONE', *, *, #2388, .F. ) ;
#8853=CARTESIAN_POINT ( 'NONE',  ( 0.4684132450478840637, -0.1062614382955253817, 0.2194422276453884824 ) ) ;
#8870=B_SPLINE_CURVE_WITH_KNOTS ( 'NONE', 3,
 ( #15452, #22061, #350, #23923, #19944, #24046, #21522, #598, #8929, #9191 ),
 .UNSPECIFIED., .F., .F.,
 ( 4, 2, 2, 2, 4 ),
 ( 0.000000000000000000, 0.2500000000000001110, 0.5000000000000002220, 0.7500000000000003331, 1.000000000000000000 ),
 .UNSPECIFIED. ) ;
#8885=EDGE_LOOP ( 'NONE', ( #15087, #20355, #8844, #5825 ) ) ;
#8892=B_SPLINE_CURVE_WITH_KNOTS ( 'NONE', 3,
 ( #16823, #14732, #14995, #20662, #12847, #16292, #2118, #1974, #10736, #12579 ),
 .UNSPECIFIED., .F., .F.,
 ( 4, 2, 2, 2, 4 ),
 ( 0.000000000000000000, 0.2499999999999998890, 0.4999999999999997780, 0.7499999999999996669, 1.000000000000000000 ),
 .UNSPECIFIED. ) ;
#8897=CARTESIAN_POINT ( 'NONE',  ( 0.4160174684701755665, 0.3320469875258716397, 0.1322810039474933141 ) ) ;
#8899=CARTESIAN_POINT ( 'NONE',  ( 0.3183792087432348872, -0.6629319518599616767, 0.2763636194390191592 ) ) ;
#8912=DIRECTION ( 'NONE',  ( 1.000000000000000000, 0.000000000000000000, 0.000000000000000000 ) ) ;
#8927=AXIS2_PLACEMENT_3D ( 'NONE', #25679, #8981, #12948 ) ;
#8929=CARTESIAN_POINT ( 'NONE',  ( 0.6867658503605201803, -0.1559616964378681969, 0.3281099440185237248 ) ) ;
#8941=CIRCLE ( 'NONE', #26515, 0.5322834645669292097 ) ;
#8949=CARTESIAN_POINT ( 'NONE',  ( 0.4158785340170984557, 0.3322209827720822850, 0.3401591244667909186 ) ) ;
#8957=EDGE_CURVE ( 'NONE', #1755, #9314, #8361, .T. ) ;
#8958=ADVANCED_FACE ( 'NONE', ( #8627 ), #8233, .F. ) ;
#8963=CARTESIAN_POINT ( 'NONE',  ( -0.2303471512294322787, -0.4798602677570401598, 0.3401574803149606252 ) ) ;
#8970=ORIENTED_EDGE ( 'NONE', *, *, #1526, .F. ) ;
#8981=DIRECTION ( 'NONE',  ( 0.000000000000000000, 0.000000000000000000, 1.000000000000000000 ) ) ;
#8989=VERTEX_POINT ( 'NONE', #15006 ) ;
#9005=FACE_OUTER_BOUND ( 'NONE', #6886, .T. ) ;
#9013=VERTEX_POINT ( 'NONE', #18037 ) ;
#9031=CARTESIAN_POINT ( 'NONE',  ( 0.0004447986960614961401, 0.5322833254990984031, 0.3401591244667909186 ) ) ;
#9049=AXIS2_PLACEMENT_3D ( 'NONE', #10830, #7010, #19445 ) ;
#9075=CARTESIAN_POINT ( 'NONE',  ( -0.0006345105826669221114, 0.4803145415259080231, 0.2194422276343239164 ) ) ;
#9077=DIRECTION ( 'NONE',  ( 0.4338837391175581204, 0.9009688679024192570, -0.000000000000000000 ) ) ;
#9081=AXIS2_PLACEMENT_3D ( 'NONE', #24752, #16007, #24461 ) ;
#9100=EDGE_LOOP ( 'NONE', ( #16327, #10744, #13790, #23170 ) ) ;
#9115=CARTESIAN_POINT ( 'NONE',  ( -0.5377323685532543474, 0.4294741335735771659, 0.3401591245381555551 ) ) ;
#9121=AXIS2_PLACEMENT_3D ( 'NONE', #12706, #27560, #6093 ) ;
#9124=EDGE_LOOP ( 'NONE', ( #23149, #2087, #10454, #5204, #27581, #11490, #20748, #695 ) ) ;
#9129=CARTESIAN_POINT ( 'NONE',  ( -0.3048711895205613587, -0.6348424542980738439, 0.3281099440176195592 ) ) ;
#9139=CARTESIAN_POINT ( 'NONE',  ( -0.0006568023596623034704, 0.5148705051068777072, 0.3251195115599746499 ) ) ;
#9142=ADVANCED_FACE ( 'NONE', ( #2940 ), #10928, .T. ) ;
#9144=CARTESIAN_POINT ( 'NONE',  ( -0.5949363243629232079, -0.1357903337134990229, 0.2362204724409449064 ) ) ;
#9163=AXIS2_PLACEMENT_3D ( 'NONE', #3188, #18008, #9699 ) ;
#9165=CARTESIAN_POINT ( 'NONE',  ( 0.000000000000000000, 0.000000000000000000, 0.4488188976377953110 ) ) ;
#9169=CARTESIAN_POINT ( 'NONE',  ( 0.4834654033848707622, -0.1110087727129997481, 0.2989974301291331016 ) ) ;
#9172=DIRECTION ( 'NONE',  ( 0.000000000000000000, 0.000000000000000000, 1.000000000000000000 ) ) ;
#9175=CARTESIAN_POINT ( 'NONE',  ( -0.4890020181336406924, -0.1109469068267769365, 0.3080453759532011393 ) ) ;
#9191=CARTESIAN_POINT ( 'NONE',  ( 0.6711032387266713251, -0.1523958994812761869, 0.3401574803149606252 ) ) ;
#9194=DIRECTION ( 'NONE',  ( 1.000000000000000000, 0.000000000000000000, 0.000000000000000000 ) ) ;
#9207=CARTESIAN_POINT ( 'NONE',  ( 0.2983664441502653641, -0.6201464311010354002, 0.3401599409343967761 ) ) ;
#9220=DIRECTION ( 'NONE',  ( 0.000000000000000000, 1.000000000000000000, 0.000000000000000000 ) ) ;
#9221=CARTESIAN_POINT ( 'NONE',  ( 0.5188885761056504231, -0.1186607836835328750, 0.1322810039474935084 ) ) ;
#9224=CARTESIAN_POINT ( 'NONE',  ( -0.2228021814306022086, -0.4641672719493093457, 0.3251195115408473946 ) ) ;
#9236=CARTESIAN_POINT ( 'NONE',  ( -0.4164331889188472857, 0.3315254675241992577, 0.1322818204150988386 ) ) ;
#9243=CARTESIAN_POINT ( 'NONE',  ( -4.821444091131312140E-17, -0.3937007874015748254, 0.4488188976377953110 ) ) ;
#9247=ORIENTED_EDGE ( 'NONE', *, *, #7229, .T. ) ;
#9253=ORIENTED_EDGE ( 'NONE', *, *, #27347, .T. ) ;
#9255=DIRECTION ( 'NONE',  ( 0.000000000000000000, 0.000000000000000000, 1.000000000000000000 ) ) ;
#9270=B_SPLINE_CURVE_WITH_KNOTS ( 'NONE', 3,
 ( #25444, #8359, #10169, #20643, #3975, #25011 ),
 .UNSPECIFIED., .F., .F.,
 ( 4, 2, 4 ),
 ( 1.217380381967462011, 1.219305002860848086, 1.221229623754231941 ),
 .UNSPECIFIED. ) ;
#9274=DIRECTION ( 'NONE',  ( -0.4338837391175581204, 0.9009688679024192570, 0.000000000000000000 ) ) ;
#9276=CARTESIAN_POINT ( 'NONE',  ( 0.4029514798603574532, 0.3205030004498418683, 0.1473214333212670424 ) ) ;
#9283=CARTESIAN_POINT ( 'NONE',  ( -0.2647715730835492609, -0.5498038367121063086, 0.2362204724409449064 ) ) ;
#9284=CARTESIAN_POINT ( 'NONE',  ( 0.6707652279343347956, -0.1538768215240155779, 0.3401574803149606252 ) ) ;
#9301=DIRECTION ( 'NONE',  ( 0.000000000000000000, 1.000000000000000000, 0.000000000000000000 ) ) ;
#9308=DIRECTION ( 'NONE',  ( 1.000000000000000000, 0.000000000000000000, 0.000000000000000000 ) ) ;
#9309=VERTEX_POINT ( 'NONE', #5646 ) ;
#9314=VERTEX_POINT ( 'NONE', #4587 ) ;
#9319=ORIENTED_EDGE ( 'NONE', *, *, #26814, .T. ) ;
#9320=EDGE_CURVE ( 'NONE', #25431, #25742, #20564, .T. ) ;
#9346=EDGE_CURVE ( 'NONE', #4356, #10683, #13656, .T. ) ;
#9351=DIRECTION ( 'NONE',  ( 0.000000000000000000, 1.000000000000000000, 0.000000000000000000 ) ) ;
#9370=ORIENTED_EDGE ( 'NONE', *, *, #10935, .F. ) ;
#9408=CARTESIAN_POINT ( 'NONE',  ( -0.2313498293151122209, -0.4793777142568558802, 0.1322818204150990051 ) ) ;
#9416=ORIENTED_EDGE ( 'NONE', *, *, #25752, .T. ) ;
#9418=CARTESIAN_POINT ( 'NONE',  ( 0.5949363243629232079, -0.1357903337134992172, 0.2362204724409449064 ) ) ;
#9420=EDGE_CURVE ( 'NONE', #2922, #20821, #23286, .T. ) ;
#9425=EDGE_LOOP ( 'NONE', ( #19568, #19081 ) ) ;
#9445=DIRECTION ( 'NONE',  ( 0.000000000000000000, -1.000000000000000000, 0.000000000000000000 ) ) ;
#9470=CARTESIAN_POINT ( 'NONE',  ( 0.2988215684303964781, -0.6199272547993208704, 0.1322810039474933141 ) ) ;
#9471=ORIENTED_EDGE ( 'NONE', *, *, #17530, .T. ) ;
#9476=EDGE_CURVE ( 'NONE', #21655, #6603, #15920, .T. ) ;
#9486=CARTESIAN_POINT ( 'NONE',  ( 0.000000000000000000, 0.6102362204724409711, 0.2362204724409449064 ) ) ;
#9524=ORIENTED_EDGE ( 'NONE', *, *, #10981, .F. ) ;
#9539=CIRCLE ( 'NONE', #9081, 0.1299212598425196763 ) ;
#9540=B_SPLINE_CURVE_WITH_KNOTS ( 'NONE', 3,
 ( #6977, #15463, #21951, #24062, #22075, #4696, #13591, #5108, #26580, #13322 ),
 .UNSPECIFIED., .F., .F.,
 ( 4, 2, 2, 2, 4 ),
 ( 0.000000000000000000, 0.2500000000000000000, 0.5000000000000000000, 0.7500000000000000000, 1.000000000000000000 ),
 .UNSPECIFIED. ) ;
#9541=CARTESIAN_POINT ( 'NONE',  ( -0.3204319178471763951, -0.6672004808837513901, 0.2562996996000485028 ) ) ;
#9550=AXIS2_PLACEMENT_3D ( 'NONE', #1527, #9860, #8039 ) ;
#9551=ORIENTED_EDGE ( 'NONE', *, *, #22970, .T. ) ;
#9555=DIRECTION ( 'NONE',  ( 0.000000000000000000, 1.000000000000000000, 0.000000000000000000 ) ) ;
#9562=DIRECTION ( 'NONE',  ( 1.000000000000000000, 0.000000000000000000, 0.000000000000000000 ) ) ;
#9566=EDGE_LOOP ( 'NONE', ( #22929, #1313 ) ) ;
#9575=B_SPLINE_CURVE_WITH_KNOTS ( 'NONE', 3,
 ( #24680, #13966, #5492, #1118, #26962, #14103 ),
 .UNSPECIFIED., .F., .F.,
 ( 4, 2, 4 ),
 ( 1.217380381967464009, 1.219305002860850085, 1.221229623754233939 ),
 .UNSPECIFIED. ) ;
#9582=CYLINDRICAL_SURFACE ( 'NONE', #21807, 0.8267716535433071723 ) ;
#9622=VECTOR ( 'NONE', #20864, 39.37007874015748143 ) ;
#9627=CARTESIAN_POINT ( 'NONE',  ( -0.2315507648392299000, -0.4792806379917101678, 0.3401574803149606252 ) ) ;
#9635=EDGE_LOOP ( 'NONE', ( #20274, #21132 ) ) ;
#9642=ORIENTED_EDGE ( 'NONE', *, *, #4507, .T. ) ;
#9664=PRODUCT_DEFINITION_CONTEXT ( 'detailed design', #22258, 'design' ) ;
#9678=VERTEX_POINT ( 'NONE', #10496 ) ;
#9699=DIRECTION ( 'NONE',  ( 1.000000000000000000, 0.000000000000000000, 0.000000000000000000 ) ) ;
#9709=DIRECTION ( 'NONE',  ( 0.9749279121818236193, -0.2225209339563147815, 0.000000000000000000 ) ) ;
#9728=CIRCLE ( 'NONE', #13337, 0.6881889763779527325 ) ;
#9734=CARTESIAN_POINT ( 'NONE',  ( 0.000000000000000000, 0.000000000000000000, 0.2362204724409449064 ) ) ;
#9745=CARTESIAN_POINT ( 'NONE',  ( -0.4173228346456693272, 5.110730736599190647E-17, 0.02362204724409448786 ) ) ;
#9746=CARTESIAN_POINT ( 'NONE',  ( -0.4713455951393992760, -0.1082342125223313134, 0.2008762816256353667 ) ) ;
#9754=SPHERICAL_SURFACE ( 'NONE', #10046, 0.1299232283464566984 ) ;
#9759=ADVANCED_FACE ( 'NONE', ( #4292 ), #21799, .F. ) ;
#9788=ORIENTED_EDGE ( 'NONE', *, *, #9346, .T. ) ;
#9798=AXIS2_PLACEMENT_3D ( 'NONE', #15973, #11867, #18344 ) ;
#9802=TOROIDAL_SURFACE ( 'NONE', #19266, 0.8031496062992127261, 0.02362204724409448786 ) ;
#9806=VERTEX_POINT ( 'NONE', #15588 ) ;
#9809=ADVANCED_FACE ( 'NONE', ( #24191, #19403 ), #10637, .T. ) ;
#9822=DIRECTION ( 'NONE',  ( 0.000000000000000000, 0.000000000000000000, 1.000000000000000000 ) ) ;
#9833=CIRCLE ( 'NONE', #24701, 0.1299212598425196763 ) ;
#9834=FACE_BOUND ( 'NONE', #3972, .T. ) ;
#9860=DIRECTION ( 'NONE',  ( 0.000000000000000000, 0.000000000000000000, 1.000000000000000000 ) ) ;
#9868=EDGE_CURVE ( 'NONE', #21006, #10381, #1647, .T. ) ;
#9874=AXIS2_PLACEMENT_3D ( 'NONE', #15077, #4966, #24318 ) ;
#9875=CIRCLE ( 'NONE', #1772, 0.6881889763779527325 ) ;
#9878=AXIS2_PLACEMENT_3D ( 'NONE', #10121, #8020, #21004 ) ;
#9905=CARTESIAN_POINT ( 'NONE',  ( 0.000000000000000000, 0.000000000000000000, 0.4488188976377953110 ) ) ;
#9917=CARTESIAN_POINT ( 'NONE',  ( -0.2311492806687369950, -0.4794744477484330636, 0.3401599409343964431 ) ) ;
#9918=EDGE_CURVE ( 'NONE', #20576, #6454, #15496, .T. ) ;
#9920=CARTESIAN_POINT ( 'NONE',  ( 0.000000000000000000, 0.5322834645669292097, 0.3401599409343964431 ) ) ;
#9924=DIRECTION ( 'NONE',  ( -0.7818314824680302477, -0.6234898018587331503, 0.000000000000000000 ) ) ;
#9928=CARTESIAN_POINT ( 'NONE',  ( -0.0007595033562148819414, 0.6881885572739390167, 0.1322834645669291320 ) ) ;
#9940=COLOUR_RGB ( '', 0.09019608, 0.27058824, 0.51372549) ;
#9953=FACE_OUTER_BOUND ( 'NONE', #8397, .T. ) ;
#9960=DIRECTION ( 'NONE',  ( 0.000000000000000000, 0.000000000000000000, 1.000000000000000000 ) ) ;
#9968=VERTEX_POINT ( 'NONE', #22064 ) ;
#9969=APPLICATION_CONTEXT ( 'automotive_design' ) ;
#9972=B_SPLINE_CURVE_WITH_KNOTS ( 'NONE', 3,
 ( #22348, #26717, #13873, #1437, #22492, #11894, #3393, #3121 ),
 .UNSPECIFIED., .F., .F.,
 ( 4, 2, 2, 4 ),
 ( 0.000000000000000000, 0.1250000000000001110, 0.2500000000000002220, 0.5000000000000000000 ),
 .UNSPECIFIED. ) ;
#9978=AXIS2_PLACEMENT_3D ( 'NONE', #2795, #2937, #17781 ) ;
#9980=CIRCLE ( 'NONE', #5948, 0.8267716535433071723 ) ;
#9988=CARTESIAN_POINT ( 'NONE',  ( -0.5949363243629232079, -0.1357903337134990229, 0.3661437007874016047 ) ) ;
#9991=FACE_OUTER_BOUND ( 'NONE', #3199, .T. ) ;
#10021=ADVANCED_FACE ( 'NONE', ( #7225 ), #1508, .F. ) ;
#10046=AXIS2_PLACEMENT_3D ( 'NONE', #15978, #8045, #21313 ) ;
#10064=TOROIDAL_SURFACE ( 'NONE', #6918, 0.6102362204724409711, 0.1299212598425196763 ) ;
#10076=ORIENTED_EDGE ( 'NONE', *, *, #1693, .T. ) ;
#10091=CARTESIAN_POINT ( 'NONE',  ( 0.5501272682997877528, 0.4396946356868946526, 0.3281099440176548088 ) ) ;
#10101=CARTESIAN_POINT ( 'NONE',  ( -0.5385210225480960844, 0.4284847435812472183, 0.1322834645669291320 ) ) ;
#10114=EDGE_CURVE ( 'NONE', #19539, #24735, #600, .T. ) ;
#10116=DIRECTION ( 'NONE',  ( 0.000000000000000000, 1.000000000000000000, 0.000000000000000000 ) ) ;
#10121=CARTESIAN_POINT ( 'NONE',  ( 0.000000000000000000, 0.000000000000000000, 0.1322834645669291320 ) ) ;
#10126=DIRECTION ( 'NONE',  ( 0.000000000000000000, 1.000000000000000000, 0.000000000000000000 ) ) ;
#10133=CARTESIAN_POINT ( 'NONE',  ( -0.4165721057576322606, 0.3313508221749649763, 0.1322834645669291320 ) ) ;
#10149=ORIENTED_EDGE ( 'NONE', *, *, #19269, .T. ) ;
#10169=CARTESIAN_POINT ( 'NONE',  ( 0.5378903297326614874, 0.4292762795476984805, 0.3401599409343964431 ) ) ;
#10175=CARTESIAN_POINT ( 'NONE',  ( 0.0006679551606482677165, 0.5322830454629158270, 0.1322834645669291320 ) ) ;
#10183=CARTESIAN_POINT ( 'NONE',  ( 0.000000000000000000, 0.000000000000000000, 0.3401574803149606252 ) ) ;
#10230=CARTESIAN_POINT ( 'NONE',  ( 0.2092582568855835823, -0.4359957531126701924, 0.2008762816647728100 ) ) ;
#10270=VERTEX_POINT ( 'NONE', #27276 ) ;
#10271=CARTESIAN_POINT ( 'NONE',  ( 0.3924375359088155268, 0.3121297331100029715, 0.1643955689165516598 ) ) ;
#10281=ORIENTED_EDGE ( 'NONE', *, *, #26237, .F. ) ;
#10315=CIRCLE ( 'NONE', #16642, 0.5322834645669292097 ) ;
#10317=CARTESIAN_POINT ( 'NONE',  ( 0.000000000000000000, 0.5322834645669292097, 0.3401599409343964431 ) ) ;
#10332=ADVANCED_FACE ( 'NONE', ( #26063 ), #13970, .T. ) ;
#10353=DIRECTION ( 'NONE',  ( 1.224646799147353207E-16, 1.000000000000000000, -0.000000000000000000 ) ) ;
#10358=B_SPLINE_CURVE_WITH_KNOTS ( 'NONE', 3,
 ( #10777, #19805, #25758, #15175, #467, #4427 ),
 .UNSPECIFIED., .F., .F.,
 ( 4, 2, 4 ),
 ( 0.4045103800602309896, 0.4064350009536160102, 0.4083596218470010308 ),
 .UNSPECIFIED. ) ;
#10373=ORIENTED_EDGE ( 'NONE', *, *, #1565, .F. ) ;
#10381=VERTEX_POINT ( 'NONE', #1385 ) ;
#10382=AXIS2_PLACEMENT_3D ( 'NONE', #4043, #20987, #3894 ) ;
#10411=ORIENTED_EDGE ( 'NONE', *, *, #2229, .F. ) ;
#10417=ORIENTED_EDGE ( 'NONE', *, *, #23604, .T. ) ;
#10434=CARTESIAN_POINT ( 'NONE',  ( -0.3924375359084866788, 0.3121297331097429018, 0.3080453759647233114 ) ) ;
#10454=ORIENTED_EDGE ( 'NONE', *, *, #14171, .F. ) ;
#10457=ORIENTED_EDGE ( 'NONE', *, *, #12047, .F. ) ;
#10496=CARTESIAN_POINT ( 'NONE',  ( 0.5375739373539409893, 0.4296723508511047229, 0.1322834645669291320 ) ) ;
#10509=DIRECTION ( 'NONE',  ( 0.6234898018587331503, -0.7818314824680301367, 0.000000000000000000 ) ) ;
#10514=DIRECTION ( 'NONE',  ( 0.000000000000000000, 0.000000000000000000, 1.000000000000000000 ) ) ;
#10550=ORIENTED_EDGE ( 'NONE', *, *, #1608, .T. ) ;
#10572=CARTESIAN_POINT ( 'NONE',  ( -0.6707652279343464530, -0.1538768215239710857, 0.1322834645669291320 ) ) ;
#10585=EDGE_CURVE ( 'NONE', #6542, #11692, #4359, .T. ) ;
#10594=CARTESIAN_POINT ( 'NONE',  ( 0.3759206409296169116, 0.2989751379763687655, 0.2362204724409450174 ) ) ;
#10599=CARTESIAN_POINT ( 'NONE',  ( 0.000000000000000000, 0.000000000000000000, 0.2362204724409449064 ) ) ;
#10601=EDGE_CURVE ( 'NONE', #23254, #12366, #12739, .T. ) ;
#10613=ORIENTED_EDGE ( 'NONE', *, *, #15491, .F. ) ;
#10637=SPHERICAL_SURFACE ( 'NONE', #26762, 0.1299232283464566984 ) ;
#10638=CARTESIAN_POINT ( 'NONE',  ( -0.2169784220115218709, -0.4520537072531055078, 0.1643955689481572668 ) ) ;
#10655=CARTESIAN_POINT ( 'NONE',  ( -0.6708219662590886312, -0.1536294932067314989, 0.3401591245381555551 ) ) ;
#10661=PRODUCT_DEFINITION_FORMATION_WITH_SPECIFIED_SOURCE ( 'ANY', '', #25836, .NOT_KNOWN. ) ;
#10681=B_SPLINE_CURVE_WITH_KNOTS ( 'NONE', 3,
 ( #8745, #17366, #11003, #6638, #23874, #17090 ),
 .UNSPECIFIED., .F., .F.,
 ( 4, 2, 4 ),
 ( 0.3864984308775630262, 0.3881911340211369743, 0.3898838371647110335 ),
 .UNSPECIFIED. ) ;
#10683=VERTEX_POINT ( 'NONE', #9243 ) ;
#10698=ORIENTED_EDGE ( 'NONE', *, *, #21675, .F. ) ;
#10736=CARTESIAN_POINT ( 'NONE',  ( 0.3062557396315260250, -0.6341756901077876263, 0.3281099440165241576 ) ) ;
#10737=EDGE_CURVE ( 'NONE', #16391, #24778, #21869, .T. ) ;
#10738=ORIENTED_EDGE ( 'NONE', *, *, #24251, .F. ) ;
#10739=EDGE_LOOP ( 'NONE', ( #10417, #5634, #20788, #11113 ) ) ;
#10740=CARTESIAN_POINT ( 'NONE',  ( 0.000000000000000000, 0.000000000000000000, 0.1322834645669291320 ) ) ;
#10744=ORIENTED_EDGE ( 'NONE', *, *, #20443, .F. ) ;
#10749=CARTESIAN_POINT ( 'NONE',  ( -0.4716287720745061529, -0.1069935333114224313, 0.2008762816207269042 ) ) ;
#10773=ORIENTED_EDGE ( 'NONE', *, *, #14373, .F. ) ;
#10777=CARTESIAN_POINT ( 'NONE',  ( -0.2992781133269515892, -0.6197069291944330427, 0.1322834645669291320 ) ) ;
#10786=ADVANCED_FACE ( 'NONE', ( #5305 ), #16193, .T. ) ;
#10792=CARTESIAN_POINT ( 'NONE',  ( 0.2315507648392299000, -0.4792806379917101678, 0.3401574803149606252 ) ) ;
#10793=CARTESIAN_POINT ( 'NONE',  ( -0.5744851493158656952, 0.4591414886146410468, 0.1960773254330283877 ) ) ;
#10802=CARTESIAN_POINT ( 'NONE',  ( 0.4173228346456693272, 0.000000000000000000, 0.4488188976377953110 ) ) ;
#10829=DIRECTION ( 'NONE',  ( 0.000000000000000000, 0.000000000000000000, 1.000000000000000000 ) ) ;
#10830=CARTESIAN_POINT ( 'NONE',  ( 0.000000000000000000, 0.000000000000000000, 0.4062992125984251635 ) ) ;
#10831=CARTESIAN_POINT ( 'NONE',  ( -0.4771018889076559244, 0.3804760601893846794, 0.3661437007874016047 ) ) ;
#10836=CARTESIAN_POINT ( 'NONE',  ( 0.5754648248638597474, 0.4579130143396930031, 0.1960773254437022384 ) ) ;
#10851=CIRCLE ( 'NONE', #24834, 0.5322834645669292097 ) ;
#10876=EDGE_LOOP ( 'NONE', ( #3519, #6345 ) ) ;
#10879=ADVANCED_FACE ( 'NONE', ( #26453 ), #26592, .T. ) ;
#10885=ADVANCED_FACE ( 'NONE', ( #8818 ), #18613, .F. ) ;
#10886=DIRECTION ( 'NONE',  ( 0.000000000000000000, -1.000000000000000000, 0.000000000000000000 ) ) ;
#10902=ORIENTED_EDGE ( 'NONE', *, *, #1628, .T. ) ;
#10915=FACE_OUTER_BOUND ( 'NONE', #20832, .T. ) ;
#10921=CARTESIAN_POINT ( 'NONE',  ( 0.2981382804008161913, -0.6202561546315472629, 0.1322818203437344520 ) ) ;
#10928=TOROIDAL_SURFACE ( 'NONE', #24451, 0.4173228346456693272, 0.02362204724409448786 ) ;
#10929=B_SPLINE_CURVE_WITH_KNOTS ( 'NONE', 3,
 ( #19963, #7381, #619, #9207, #13882, #24605 ),
 .UNSPECIFIED., .F., .F.,
 ( 4, 2, 4 ),
 ( 1.217380381967462011, 1.219305002860848086, 1.221229623754233939 ),
 .UNSPECIFIED. ) ;
#10931=CARTESIAN_POINT ( 'NONE',  ( -0.5604501195207933772, 0.4479362078532184155, 0.1601585119423933334 ) ) ;
#10935=EDGE_CURVE ( 'NONE', #25110, #19539, #17701, .T. ) ;
#10949=CARTESIAN_POINT ( 'NONE',  ( 0.5189874374926378708, -0.1182276436463391700, 0.1322810039474935084 ) ) ;
#10955=DIRECTION ( 'NONE',  ( 0.000000000000000000, -1.000000000000000000, 0.000000000000000000 ) ) ;
#10957=CARTESIAN_POINT ( 'NONE',  ( -0.6711032387266713251, -0.1523958994812759926, 0.3401574803149606252 ) ) ;
#10960=EDGE_CURVE ( 'NONE', #23531, #23608, #27575, .T. ) ;
#10966=CARTESIAN_POINT ( 'NONE',  ( 0.5021077788563528266, -0.1139291307083610677, 0.3251195115536875124 ) ) ;
#10973=CIRCLE ( 'NONE', #25415, 0.4173228346456693272 ) ;
#10981=EDGE_CURVE ( 'NONE', #4492, #14265, #24926, .T. ) ;
#11000=CARTESIAN_POINT ( 'NONE',  ( -0.0006345105826669216777, 0.4803145415259080786, 0.2529987172475652857 ) ) ;
#11003=CARTESIAN_POINT ( 'NONE',  ( -0.5188885761056504231, -0.1186607836835326668, 0.1322810039474935084 ) ) ;
#11005=FILL_AREA_STYLE_COLOUR ( '', #9940 ) ;
#11015=TOROIDAL_SURFACE ( 'NONE', #26791, 0.6102362204724409711, 0.1299212598425196763 ) ;
#11017=CARTESIAN_POINT ( 'NONE',  ( 0.7168072604734050390, -0.1644124225522937965, 0.2763636194388741085 ) ) ;
#11048=CARTESIAN_POINT ( 'NONE',  ( 0.000000000000000000, 0.000000000000000000, -1.092739370078740131E-17 ) ) ;
#11070=DIRECTION ( 'NONE',  ( 0.000000000000000000, 1.000000000000000000, 0.000000000000000000 ) ) ;
#11077=B_SPLINE_CURVE_WITH_KNOTS ( 'NONE', 3,
 ( #2192, #6577, #10949, #9221, #19574, #19707 ),
 .UNSPECIFIED., .F., .F.,
 ( 4, 2, 4 ),
 ( 0.3864984308775630262, 0.3881911340211369743, 0.3898838371647110335 ),
 .UNSPECIFIED. ) ;
#11078=ORIENTED_EDGE ( 'NONE', *, *, #5935, .F. ) ;
#11099=ADVANCED_FACE ( 'NONE', ( #24757 ), #18668, .T. ) ;
#11102=EDGE_LOOP ( 'NONE', ( #4986, #22313, #12064, #24382, #24667, #12211 ) ) ;
#11104=CARTESIAN_POINT ( 'NONE',  ( 0.000000000000000000, 0.000000000000000000, 0.1322834645669291320 ) ) ;
#11113=ORIENTED_EDGE ( 'NONE', *, *, #11181, .F. ) ;
#11115=DIRECTION ( 'NONE',  ( 0.000000000000000000, 1.000000000000000000, 0.000000000000000000 ) ) ;
#11120=CARTESIAN_POINT ( 'NONE',  ( 0.3937007874015748254, 0.000000000000000000, 0.02362204724409448786 ) ) ;
#11121=ORIENTED_EDGE ( 'NONE', *, *, #6972, .F. ) ;
#11139=CARTESIAN_POINT ( 'NONE',  ( 0.0006443779181942713890, 0.4960456921234573935, 0.1734435147384566500 ) ) ;
#11142=VERTEX_POINT ( 'NONE', #12185 ) ;
#11147=DIRECTION ( 'NONE',  ( -0.9009688679024190350, 0.4338837391175582314, 0.000000000000000000 ) ) ;
#11156=DIRECTION ( 'NONE',  ( 0.000000000000000000, -1.000000000000000000, 0.000000000000000000 ) ) ;
#11161=CARTESIAN_POINT ( 'NONE',  ( 0.3204319178470658724, -0.6672004808835035883, 0.2562996996018049312 ) ) ;
#11176=ORIENTED_EDGE ( 'NONE', *, *, #4865, .T. ) ;
#11179=DIRECTION ( 'NONE',  ( 0.000000000000000000, -1.000000000000000000, 0.000000000000000000 ) ) ;
#11181=EDGE_CURVE ( 'NONE', #1421, #26488, #5063, .T. ) ;
#11182=CARTESIAN_POINT ( 'NONE',  ( 0.000000000000000000, 0.000000000000000000, 0.2362204724409449064 ) ) ;
#11196=CARTESIAN_POINT ( 'NONE',  ( 7.955503286468943460E-18, 0.6102362204724409711, 0.3661437007874016047 ) ) ;
#11207=DIRECTION ( 'NONE',  ( 0.000000000000000000, 0.000000000000000000, 1.000000000000000000 ) ) ;
#11216=CARTESIAN_POINT ( 'NONE',  ( 0.000000000000000000, 0.000000000000000000, 0.06614173228346456601 ) ) ;
#11234=CARTESIAN_POINT ( 'NONE',  ( 0.4157391792961063204, 0.3323952789219082882, 0.3401574803149606252 ) ) ;
#11248=CARTESIAN_POINT ( 'NONE',  ( -0.5382052855068000241, 0.4288813374988101890, 0.3401599409343964431 ) ) ;
#11251=ORIENTED_EDGE ( 'NONE', *, *, #11538, .F. ) ;
#11259=VERTEX_POINT ( 'NONE', #17274 ) ;
#11266=CARTESIAN_POINT ( 'NONE',  ( -0.2979095355689177493, -0.6203660015065670663, 0.3401574803149606252 ) ) ;
#11269=EDGE_CURVE ( 'NONE', #27077, #22659, #24948, .T. ) ;
#11285=ORIENTED_EDGE ( 'NONE', *, *, #20791, .F. ) ;
#11291=VERTEX_POINT ( 'NONE', #24040 ) ;
#11301=DIRECTION ( 'NONE',  ( 0.000000000000000000, 1.000000000000000000, 0.000000000000000000 ) ) ;
#11308=DIRECTION ( 'NONE',  ( 0.000000000000000000, 1.000000000000000000, 0.000000000000000000 ) ) ;
#11320=DIRECTION ( 'NONE',  ( 1.000000000000000000, 0.000000000000000000, 0.000000000000000000 ) ) ;
#11339=CARTESIAN_POINT ( 'NONE',  ( 0.000000000000000000, 0.000000000000000000, 0.2362204724409449064 ) ) ;
#11347=CARTESIAN_POINT ( 'NONE',  ( 0.000000000000000000, 0.000000000000000000, 0.02362204724409448786 ) ) ;
#11348=CARTESIAN_POINT ( 'NONE',  ( 0.2303471512294322787, -0.4798602677570401598, 0.1322834645669291320 ) ) ;
#11353=CARTESIAN_POINT ( 'NONE',  ( 0.4771018889076559244, 0.3804760601893846794, 0.2362204724409449064 ) ) ;
#11357=ORIENTED_EDGE ( 'NONE', *, *, #12974, .T. ) ;
#11374=LINE ( 'NONE', #4732, #12398 ) ;
#11378=ADVANCED_FACE ( 'NONE', ( #6501 ), #10064, .F. ) ;
#11391=VERTEX_POINT ( 'NONE', #2312 ) ;
#11410=DIRECTION ( 'NONE',  ( -0.2225209339563143096, 0.9749279121818237304, 0.000000000000000000 ) ) ;
#11411=ADVANCED_FACE ( 'NONE', ( #22084, #758 ), #9754, .T. ) ;
#11422=VERTEX_POINT ( 'NONE', #728 ) ;
#11425=VERTEX_POINT ( 'NONE', #8321 ) ;
#11434=CARTESIAN_POINT ( 'NONE',  ( -0.4021324607134745821, 0.3215300179743675324, 0.3251195115596967611 ) ) ;
#11436=DIRECTION ( 'NONE',  ( 0.000000000000000000, 0.000000000000000000, -1.000000000000000000 ) ) ;
#11438=DIRECTION ( 'NONE',  ( 1.000000000000000000, 0.000000000000000000, 0.000000000000000000 ) ) ;
#11487=( NAMED_UNIT ( * ) SI_UNIT ( $, .STERADIAN. ) SOLID_ANGLE_UNIT ( ) ) ;
#11489=CARTESIAN_POINT ( 'NONE',  ( 0.4165721057576322606, 0.3313508221749649763, 0.3401574803149606252 ) ) ;
#11490=ORIENTED_EDGE ( 'NONE', *, *, #21044, .F. ) ;
#11492=ORIENTED_EDGE ( 'NONE', *, *, #18272, .T. ) ;
#11493=ORIENTED_EDGE ( 'NONE', *, *, #10737, .F. ) ;
#11500=CARTESIAN_POINT ( 'NONE',  ( 0.000000000000000000, 0.000000000000000000, -1.092739370078740131E-17 ) ) ;
#11501=CIRCLE ( 'NONE', #8356, 0.4803149606299212393 ) ;
#11508=VERTEX_POINT ( 'NONE', #2631 ) ;
#11509=CIRCLE ( 'NONE', #27307, 0.8031496062992127261 ) ;
#11524=FACE_OUTER_BOUND ( 'NONE', #18595, .T. ) ;
#11538=EDGE_CURVE ( 'NONE', #1564, #2742, #13211, .T. ) ;
#11543=CARTESIAN_POINT ( 'NONE',  ( -0.6864238947227671028, -0.1574599019768544161, 0.1443310008632313346 ) ) ;
#11544=CARTESIAN_POINT ( 'NONE',  ( 0.000000000000000000, 0.000000000000000000, -1.092739370078740131E-17 ) ) ;
#11588=AXIS2_PLACEMENT_3D ( 'NONE', #5229, #3665, #7923 ) ;
#11640=CARTESIAN_POINT ( 'NONE',  ( -0.2315507648392299000, -0.4792806379917101678, 0.1322834645669291320 ) ) ;
#11641=CARTESIAN_POINT ( 'NONE',  ( -0.0006620872580285327904, 0.5229309616564024044, 0.1392975274218142823 ) ) ;
#11658=EDGE_LOOP ( 'NONE', ( #22526, #10149, #22165, #12741, #21580 ) ) ;
#11663=VERTEX_POINT ( 'NONE', #11120 ) ;
#11667=B_SPLINE_CURVE_WITH_KNOTS ( 'NONE', 3,
 ( #4740, #4484, #21988, #13362, #23843, #13224, #10836, #143, #6879, #17605 ),
 .UNSPECIFIED., .F., .F.,
 ( 4, 2, 2, 2, 4 ),
 ( 0.000000000000000000, 0.2500000000000000000, 0.5000000000000000000, 0.7500000000000000000, 1.000000000000000000 ),
 .UNSPECIFIED. ) ;
#11682=CARTESIAN_POINT ( 'NONE',  ( -0.6993003464527065560, -0.1604063846361034051, 0.1601585119460832707 ) ) ;
#11692=VERTEX_POINT ( 'NONE', #26780 ) ;
#11703=ORIENTED_EDGE ( 'NONE', *, *, #7366, .F. ) ;
#11714=CARTESIAN_POINT ( 'NONE',  ( -0.4084310843265718804, 0.3265597623311254916, 0.3331434174597265874 ) ) ;
#11722=CARTESIAN_POINT ( 'NONE',  ( 0.2228021814283700774, -0.4641672719447021422, 0.3251195115356099175 ) ) ;
#11731=ORIENTED_EDGE ( 'NONE', *, *, #14957, .F. ) ;
#11732=CARTESIAN_POINT ( 'NONE',  ( 0.000000000000000000, 0.000000000000000000, -1.092739370078740131E-17 ) ) ;
#11739=ORIENTED_EDGE ( 'NONE', *, *, #5914, .F. ) ;
#11758=DIRECTION ( 'NONE',  ( 0.000000000000000000, 0.000000000000000000, 1.000000000000000000 ) ) ;
#11783=CARTESIAN_POINT ( 'NONE',  ( 0.5949363243629232079, -0.1357903337134992172, 0.3661437007874016047 ) ) ;
#11787=AXIS2_PLACEMENT_3D ( 'NONE', #27186, #10353, #18540 ) ;
#11797=ADVANCED_FACE ( 'NONE', ( #11524 ), #4090, .T. ) ;
#11813=PLANE ( 'NONE',  #17162 ) ;
#11821=CARTESIAN_POINT ( 'NONE',  ( 0.5187889641967551313, -0.1190953285357214675, 0.3401574803149606252 ) ) ;
#11824=CARTESIAN_POINT ( 'NONE',  ( -0.6864238947242438105, -0.1574599019772051633, 0.3281099440175202497 ) ) ;
#11838=FACE_OUTER_BOUND ( 'NONE', #21591, .T. ) ;
#11846=ORIENTED_EDGE ( 'NONE', *, *, #7388, .T. ) ;
#11853=EDGE_CURVE ( 'NONE', #11391, #15542, #15399, .T. ) ;
#11855=CARTESIAN_POINT ( 'NONE',  ( 0.4165721057576322606, 0.3313508221749649763, 0.3401574803149606252 ) ) ;
#11859=DIRECTION ( 'NONE',  ( 0.000000000000000000, 0.000000000000000000, 1.000000000000000000 ) ) ;
#11860=PLANE ( 'NONE',  #7856 ) ;
#11865=CARTESIAN_POINT ( 'NONE',  ( -0.3777066424200924422, 0.3020248451651783017, 0.2008762815972411353 ) ) ;
#11867=DIRECTION ( 'NONE',  ( 0.000000000000000000, 0.000000000000000000, 1.000000000000000000 ) ) ;
#11886=CARTESIAN_POINT ( 'NONE',  ( 0.2990496115118929099, -0.6198172806991221195, 0.1322818203437344520 ) ) ;
#11894=CARTESIAN_POINT ( 'NONE',  ( -0.4713455951419531220, -0.1082342125229185797, 0.2715646632656424919 ) ) ;
#11896=FACE_OUTER_BOUND ( 'NONE', #14864, .T. ) ;
#11901=CARTESIAN_POINT ( 'NONE',  ( 0.000000000000000000, 0.000000000000000000, 0.3401574803149606252 ) ) ;
#11927=CARTESIAN_POINT ( 'NONE',  ( -0.2315507648392299000, -0.4792806379917101678, 0.1322834645669291320 ) ) ;
#11937=VERTEX_POINT ( 'NONE', #23266 ) ;
#11944=ORIENTED_EDGE ( 'NONE', *, *, #1539, .T. ) ;
#11959=FACE_BOUND ( 'NONE', #8549, .T. ) ;
#11963=CARTESIAN_POINT ( 'NONE',  ( 0.000000000000000000, 0.000000000000000000, 0.4488188976377953110 ) ) ;
#11995=AXIS2_PLACEMENT_3D ( 'NONE', #17297, #10514, #4449 ) ;
#12002=CARTESIAN_POINT ( 'NONE',  ( -0.4092566936335077510, 0.3255244810064202854, 0.3331434174600059750 ) ) ;
#12005=DIRECTION ( 'NONE',  ( 1.000000000000000000, 0.000000000000000000, 0.000000000000000000 ) ) ;
#12047=EDGE_CURVE ( 'NONE', #4395, #5951, #2983, .T. ) ;
#12064=ORIENTED_EDGE ( 'NONE', *, *, #9346, .F. ) ;
#12069=ORIENTED_EDGE ( 'NONE', *, *, #13300, .T. ) ;
#12071=EDGE_CURVE ( 'NONE', #25742, #24495, #14936, .T. ) ;
#12078=ORIENTED_EDGE ( 'NONE', *, *, #16004, .F. ) ;
#12085=EDGE_CURVE ( 'NONE', #10381, #7546, #19865, .T. ) ;
#12090=ORIENTED_EDGE ( 'NONE', *, *, #14446, .T. ) ;
#12101=CARTESIAN_POINT ( 'NONE',  ( 0.000000000000000000, 0.000000000000000000, 0.02362204724409448786 ) ) ;
#12108=MANIFOLD_SOLID_BREP ( 'Deep Groove Ball Bearing 20x42x12', #1971 ) ;
#12113=CIRCLE ( 'NONE', #15728, 0.5322834645669292097 ) ;
#12124=ORIENTED_EDGE ( 'NONE', *, *, #1474, .T. ) ;
#12129=CARTESIAN_POINT ( 'NONE',  ( -6.518592411209533944E-17, -0.5322834645669292097, 0.3401574803149606252 ) ) ;
#12185=CARTESIAN_POINT ( 'NONE',  ( -0.5187889641967551313, -0.1190953285357212593, 0.1322834645669291320 ) ) ;
#12196=DIRECTION ( 'NONE',  ( 1.000000000000000000, 0.000000000000000000, 0.000000000000000000 ) ) ;
#12211=ORIENTED_EDGE ( 'NONE', *, *, #12829, .F. ) ;
#12212=ADVANCED_FACE ( 'NONE', ( #12941 ), #15091, .F. ) ;
#12214=B_SPLINE_CURVE_WITH_KNOTS ( 'NONE', 3,
 ( #13995, #7081, #9746, #15700, #2682, #24172, #13424, #13565 ),
 .UNSPECIFIED., .F., .F.,
 ( 4, 2, 2, 4 ),
 ( 0.5000000000000000000, 0.7499999999999997780, 0.8749999999999998890, 1.000000000000000000 ),
 .UNSPECIFIED. ) ;
#12215=CARTESIAN_POINT ( 'NONE',  ( 0.5604501195244573353, 0.4479362078561491822, 0.3122824329334484283 ) ) ;
#12230=LINE ( 'NONE', #26398, #18006 ) ;
#12236=CIRCLE ( 'NONE', #11787, 0.02362204724409448092 ) ;
#12252=ORIENTED_EDGE ( 'NONE', *, *, #16658, .F. ) ;
#12256=EDGE_LOOP ( 'NONE', ( #4491, #23321, #15253, #5381 ) ) ;
#12257=CARTESIAN_POINT ( 'NONE',  ( 0.3785000865561056194, 0.3010298976871484400, 0.2008762816001854468 ) ) ;
#12292=ORIENTED_EDGE ( 'NONE', *, *, #1538, .F. ) ;
#12300=CIRCLE ( 'NONE', #23147, 0.6881889763779527325 ) ;
#12314=B_SPLINE_CURVE_WITH_KNOTS ( 'NONE', 3,
 ( #299, #19754, #23731, #26112, #422, #24259 ),
 .UNSPECIFIED., .F., .F.,
 ( 4, 2, 4 ),
 ( 1.162880698919835920, 1.164573402063409979, 1.166266105206984038 ),
 .UNSPECIFIED. ) ;
#12320=ADVANCED_FACE ( 'NONE', ( #14214 ), #27585, .F. ) ;
#12321=PRESENTATION_STYLE_ASSIGNMENT (( #3994 ) ) ;
#12333=AXIS2_PLACEMENT_3D ( 'NONE', #9905, #16978, #25304 ) ;
#12354=ORIENTED_EDGE ( 'NONE', *, *, #7891, .T. ) ;
#12363=CARTESIAN_POINT ( 'NONE',  ( 0.2262947209289010442, -0.4714317853940108716, 0.1392975274349756987 ) ) ;
#12364=CARTESIAN_POINT ( 'NONE',  ( -0.5383630292499967940, 0.4286833100733401514, 0.1322818203437346463 ) ) ;
#12366=VERTEX_POINT ( 'NONE', #2881 ) ;
#12373=ORIENTED_EDGE ( 'NONE', *, *, #22284, .T. ) ;
#12398=VECTOR ( 'NONE', #26763, 39.37007874015748143 ) ;
#12446=ORIENTED_EDGE ( 'NONE', *, *, #16486, .T. ) ;
#12464=ORIENTED_EDGE ( 'NONE', *, *, #23719, .T. ) ;
#12481=CARTESIAN_POINT ( 'NONE',  ( 0.2315507648392299000, -0.4792806379917101678, 0.3401574803149606252 ) ) ;
#12488=ORIENTED_EDGE ( 'NONE', *, *, #4655, .F. ) ;
#12493=EDGE_CURVE ( 'NONE', #22690, #17082, #9980, .T. ) ;
#12507=CARTESIAN_POINT ( 'NONE',  ( 0.2169784220059887692, -0.4520537072416159208, 0.1643955689668546716 ) ) ;
#12529=ORIENTED_EDGE ( 'NONE', *, *, #18189, .T. ) ;
#12553=CIRCLE ( 'NONE', #1774, 0.6881889763779527325 ) ;
#12559=DIRECTION ( 'NONE',  ( 0.000000000000000000, 0.000000000000000000, -1.000000000000000000 ) ) ;
#12578=ORIENTED_EDGE ( 'NONE', *, *, #2388, .T. ) ;
#12579=CARTESIAN_POINT ( 'NONE',  ( 0.2992781133269515892, -0.6197069291944330427, 0.3401574803149606252 ) ) ;
#12592=ADVANCED_FACE ( 'NONE', ( #9953 ), #15843, .F. ) ;
#12597=TOROIDAL_SURFACE ( 'NONE', #883, 0.6102362204724409711, 0.1299212598425196763 ) ;
#12608=CIRCLE ( 'NONE', #19816, 0.4803149606299212393 ) ;
#12609=CARTESIAN_POINT ( 'NONE',  ( 0.000000000000000000, 0.000000000000000000, 0.2362204724409449064 ) ) ;
#12661=CIRCLE ( 'NONE', #18026, 0.1299232283464567261 ) ;
#12662=ADVANCED_FACE ( 'NONE', ( #6982, #6705 ), #13329, .T. ) ;
#12706=CARTESIAN_POINT ( 'NONE',  ( 0.000000000000000000, 0.000000000000000000, 0.02362204724409448786 ) ) ;
#12712=CARTESIAN_POINT ( 'NONE',  ( 0.0007882571242861507056, 0.7401570605739641318, 0.2562996995998030880 ) ) ;
#12715=DIRECTION ( 'NONE',  ( 0.000000000000000000, 0.000000000000000000, -1.000000000000000000 ) ) ;
#12723=CARTESIAN_POINT ( 'NONE',  ( -0.6711032387266614441, -0.1523958994813200962, 0.1322834645669291320 ) ) ;
#12724=B_SPLINE_CURVE_WITH_KNOTS ( 'NONE', 3,
 ( #9284, #2661, #26669, #11017, #5058, #17510, #26129, #7187, #15806, #4645 ),
 .UNSPECIFIED., .F., .F.,
 ( 4, 2, 2, 2, 4 ),
 ( 0.000000000000000000, 0.2500000000000000000, 0.5000000000000000000, 0.7500000000000000000, 1.000000000000000000 ),
 .UNSPECIFIED. ) ;
#12725=CIRCLE ( 'NONE', #153, 0.8267716535433071723 ) ;
#12729=EDGE_CURVE ( 'NONE', #13999, #8723, #9539, .T. ) ;
#12733=CARTESIAN_POINT ( 'NONE',  ( 0.4173228346456693272, 0.000000000000000000, 0.4724409448818898127 ) ) ;
#12739=CIRCLE ( 'NONE', #16352, 0.5322834645669292097 ) ;
#12741=ORIENTED_EDGE ( 'NONE', *, *, #2389, .T. ) ;
#12747=CARTESIAN_POINT ( 'NONE',  ( 0.4681308612729634389, -0.1074986424507603650, 0.2194422276442969111 ) ) ;
#12754=EDGE_CURVE ( 'NONE', #21440, #11663, #536, .T. ) ;
#12764=CARTESIAN_POINT ( 'NONE',  ( -0.2146455952193271344, -0.4472013107423940537, 0.1734435147757991957 ) ) ;
#12793=CARTESIAN_POINT ( 'NONE',  ( 0.4173228346456693272, 0.000000000000000000, 0.02362204724409448786 ) ) ;
#12803=CARTESIAN_POINT ( 'NONE',  ( -0.7217751814613770911, -0.1639319465203265547, 0.2161412452679343787 ) ) ;
#12829=EDGE_CURVE ( 'NONE', #11663, #8989, #13178, .T. ) ;
#12834=DIRECTION ( 'NONE',  ( -0.9009688679024190350, -0.4338837391175581759, 0.000000000000000000 ) ) ;
#12847=CARTESIAN_POINT ( 'NONE',  ( 0.3218523081042760081, -0.6665164569853854193, 0.2161412452716660326 ) ) ;
#12851=FACE_BOUND ( 'NONE', #9124, .T. ) ;
#12855=AXIS2_PLACEMENT_3D ( 'NONE', #22569, #7884, #9555 ) ;
#12861=CARTESIAN_POINT ( 'NONE',  ( 0.4162944719209874522, 0.3316996361851579089, 0.1322810039474933141 ) ) ;
#12882=DIRECTION ( 'NONE',  ( 0.000000000000000000, 0.000000000000000000, 1.000000000000000000 ) ) ;
#12890=ORIENTED_EDGE ( 'NONE', *, *, #5935, .T. ) ;
#12941=FACE_OUTER_BOUND ( 'NONE', #7930, .T. ) ;
#12948=DIRECTION ( 'NONE',  ( 0.000000000000000000, 1.000000000000000000, 0.000000000000000000 ) ) ;
#12960=ORIENTED_EDGE ( 'NONE', *, *, #14743, .F. ) ;
#12974=EDGE_CURVE ( 'NONE', #22865, #25110, #12725, .T. ) ;
#12993=DIRECTION ( 'NONE',  ( 0.000000000000000000, -1.000000000000000000, 0.000000000000000000 ) ) ;
#13030=DIRECTION ( 'NONE',  ( 0.000000000000000000, -1.000000000000000000, 0.000000000000000000 ) ) ;
#13046=CIRCLE ( 'NONE', #18423, 0.5322834645669292097 ) ;
#13058=DIRECTION ( 'NONE',  ( 0.000000000000000000, 1.000000000000000000, 0.000000000000000000 ) ) ;
#13069=CARTESIAN_POINT ( 'NONE',  ( -8.427884271297532088E-17, -0.6881889763779527325, 0.4724409448818898127 ) ) ;
#13074=CARTESIAN_POINT ( 'NONE',  ( -0.2146455952181789972, -0.4472013107399995802, 0.2989974301012601199 ) ) ;
#13108=CARTESIAN_POINT ( 'NONE',  ( -0.3048711895200191258, -0.6348424542969446360, 0.1443310008633306996 ) ) ;
#13129=CARTESIAN_POINT ( 'NONE',  ( 0.0007756954652704383529, 0.7174612052789276495, 0.3122824329332504201 ) ) ;
#13150=DIRECTION ( 'NONE',  ( 0.000000000000000000, 0.000000000000000000, 1.000000000000000000 ) ) ;
#13154=VERTEX_POINT ( 'NONE', #6446 ) ;
#13178=CIRCLE ( 'NONE', #9121, 0.3937007874015748254 ) ;
#13180=CARTESIAN_POINT ( 'NONE',  ( -0.2647715730835492609, -0.5498038367121063086, 0.2362204724409449064 ) ) ;
#13211=CIRCLE ( 'NONE', #22227, 0.6881889763779527325 ) ;
#13224=CARTESIAN_POINT ( 'NONE',  ( 0.5791695622058307125, 0.4608640948054552045, 0.2161412452810388962 ) ) ;
#13260=B_SPLINE_CURVE_WITH_KNOTS ( 'NONE', 3,
 ( #9627, #27298, #9917, #27023, #23072, #5258 ),
 .UNSPECIFIED., .F., .F.,
 ( 4, 2, 4 ),
 ( 1.162880698919837918, 1.164573402063409979, 1.166266105206986037 ),
 .UNSPECIFIED. ) ;
#13292=TOROIDAL_SURFACE ( 'NONE', #242, 0.6102362204724409711, 0.1299212598425196763 ) ;
#13297=CARTESIAN_POINT ( 'NONE',  ( -0.5021077788565687650, -0.1139291307084100563, 0.3251195115539141645 ) ) ;
#13300=EDGE_CURVE ( 'NONE', #11508, #25524, #12300, .T. ) ;
#13318=AXIS2_PLACEMENT_3D ( 'NONE', #5630, #1523, #3341 ) ;
#13319=CARTESIAN_POINT ( 'NONE',  ( 0.000000000000000000, 0.000000000000000000, 0.1322834645669291320 ) ) ;
#13322=CARTESIAN_POINT ( 'NONE',  ( -0.5385210225480960844, 0.4284847435812472183, 0.3401574803149606252 ) ) ;
#13323=CARTESIAN_POINT ( 'NONE',  ( -0.5501272683015652198, 0.4396946356883123519, 0.3281099440159496172 ) ) ;
#13324=AXIS2_PLACEMENT_3D ( 'NONE', #5264, #11758, #22504 ) ;
#13329=SPHERICAL_SURFACE ( 'NONE', #13601, 0.1299232283464566984 ) ;
#13334=CARTESIAN_POINT ( 'NONE',  ( 0.000000000000000000, 0.000000000000000000, 0.3401574803149606252 ) ) ;
#13336=CARTESIAN_POINT ( 'NONE',  ( 0.4164331889188472857, 0.3315254675241992577, 0.3401591244667909186 ) ) ;
#13337=AXIS2_PLACEMENT_3D ( 'NONE', #13334, #11207, #19829 ) ;
#13354=ORIENTED_EDGE ( 'NONE', *, *, #3968, .T. ) ;
#13358=EDGE_CURVE ( 'NONE', #25578, #17014, #9972, .T. ) ;
#13362=CARTESIAN_POINT ( 'NONE',  ( 0.5754648248631183405, 0.4579130143391036412, 0.2763636194408833902 ) ) ;
#13383=DIRECTION ( 'NONE',  ( 0.000000000000000000, 1.000000000000000000, 0.000000000000000000 ) ) ;
#13392=( NAMED_UNIT ( * ) SI_UNIT ( $, .STERADIAN. ) SOLID_ANGLE_UNIT ( ) ) ;
#13401=ORIENTED_EDGE ( 'NONE', *, *, #1538, .T. ) ;
#13404=ORIENTED_EDGE ( 'NONE', *, *, #19269, .F. ) ;
#13407=CARTESIAN_POINT ( 'NONE',  ( -7.279147705782180972E-18, 0.5322834645669292097, 0.1322810039474933141 ) ) ;
#13424=CARTESIAN_POINT ( 'NONE',  ( -0.5096726623812283252, -0.1170085733290669172, 0.1392975274269444008 ) ) ;
#13442=VERTEX_POINT ( 'NONE', #12733 ) ;
#13514=CIRCLE ( 'NONE', #17144, 0.8267716535433071723 ) ;
#13555=CARTESIAN_POINT ( 'NONE',  ( 0.000000000000000000, 0.000000000000000000, 0.2362204724409449064 ) ) ;
#13564=CARTESIAN_POINT ( 'NONE',  ( -0.4837521785369528482, -0.1097523286760773431, 0.2989974301286330571 ) ) ;
#13565=CARTESIAN_POINT ( 'NONE',  ( -0.5187889641967551313, -0.1190953285357212593, 0.1322834645669291320 ) ) ;
#13582=ORIENTED_EDGE ( 'NONE', *, *, #4808, .T. ) ;
#13591=CARTESIAN_POINT ( 'NONE',  ( -0.5754648248646618836, 0.4579130143403264963, 0.2763636194352788178 ) ) ;
#13601=AXIS2_PLACEMENT_3D ( 'NONE', #4166, #19272, #15058 ) ;
#13607=EDGE_CURVE ( 'NONE', #22651, #5888, #5574, .T. ) ;
#13611=CARTESIAN_POINT ( 'NONE',  ( 0.2979095355690402069, -0.6203660015065080024, 0.1322834645669291320 ) ) ;
#13614=ADVANCED_FACE ( 'NONE', ( #15434 ), #24957, .F. ) ;
#13628=DIRECTION ( 'NONE',  ( 0.000000000000000000, 0.000000000000000000, 1.000000000000000000 ) ) ;
#13656=CIRCLE ( 'NONE', #3740, 0.3937007874015748254 ) ;
#13668=CARTESIAN_POINT ( 'NONE',  ( 0.2647715730835492609, -0.5498038367121063086, 0.2362204724409449064 ) ) ;
#13673=AXIS2_PLACEMENT_3D ( 'NONE', #11339, #22634, #19957 ) ;
#13684=CARTESIAN_POINT ( 'NONE',  ( 0.4029514798610943083, 0.3205030004504269003, 0.3251195115615853615 ) ) ;
#13692=CARTESIAN_POINT ( 'NONE',  ( 0.4887136534576805857, -0.1122103150229257218, 0.3080453759536327385 ) ) ;
#13697=DIRECTION ( 'NONE',  ( 0.000000000000000000, 0.000000000000000000, -1.000000000000000000 ) ) ;
#13714=FACE_OUTER_BOUND ( 'NONE', #21790, .T. ) ;
#13731=DIRECTION ( 'NONE',  ( 0.000000000000000000, 1.000000000000000000, 0.000000000000000000 ) ) ;
#13744=ORIENTED_EDGE ( 'NONE', *, *, #13607, .T. ) ;
#13757=DIRECTION ( 'NONE',  ( 0.000000000000000000, 0.000000000000000000, 1.000000000000000000 ) ) ;
#13758=CIRCLE ( 'NONE', #5179, 0.3937007874015748254 ) ;
#13765=EDGE_CURVE ( 'NONE', #13442, #5702, #10973, .T. ) ;
#13767=TOROIDAL_SURFACE ( 'NONE', #3851, 0.6102362204724409711, 0.1299212598425196763 ) ;
#13790=ORIENTED_EDGE ( 'NONE', *, *, #16486, .F. ) ;
#13798=DIRECTION ( 'NONE',  ( 0.000000000000000000, 1.000000000000000000, 0.000000000000000000 ) ) ;
#13803=CARTESIAN_POINT ( 'NONE',  ( -0.0006345105826668660581, 0.4803145415259079121, 0.2362204724409446843 ) ) ;
#13809=CARTESIAN_POINT ( 'NONE',  ( -0.7168072604723305652, -0.1644124225520415539, 0.1960773254398737175 ) ) ;
#13813=AXIS2_PLACEMENT_3D ( 'NONE', #10740, #14736, #17099 ) ;
#13825=VERTEX_POINT ( 'NONE', #7204 ) ;
#13837=DIRECTION ( 'NONE',  ( 0.000000000000000000, -1.000000000000000000, 0.000000000000000000 ) ) ;
#13840=CARTESIAN_POINT ( 'NONE',  ( 0.5187889641967551313, -0.1190953285357214675, 0.3401574803149606252 ) ) ;
#13843=UNCERTAINTY_MEASURE_WITH_UNIT (LENGTH_MEASURE( 1.000000000000000082E-05 ), #21076, 'distance_accuracy_value', 'NONE') ;
#13846=FACE_OUTER_BOUND ( 'NONE', #10876, .T. ) ;
#13847=DIRECTION ( 'NONE',  ( 0.000000000000000000, 0.000000000000000000, 1.000000000000000000 ) ) ;
#13863=B_SPLINE_CURVE_WITH_KNOTS ( 'NONE', 3,
 ( #25973, #13108, #24523, #24124, #24253, #9541, #17748, #20293, #9129, #11266 ),
 .UNSPECIFIED., .F., .F.,
 ( 4, 2, 2, 2, 4 ),
 ( 0.000000000000000000, 0.2499999999999998890, 0.4999999999999997780, 0.7499999999999996669, 1.000000000000000000 ),
 .UNSPECIFIED. ) ;
#13873=CARTESIAN_POINT ( 'NONE',  ( -0.5018154743073831581, -0.1152098006147909692, 0.3251195115537083846 ) ) ;
#13882=CARTESIAN_POINT ( 'NONE',  ( 0.2981382804007346454, -0.6202561546315846774, 0.3401591245381555551 ) ) ;
#13926=CARTESIAN_POINT ( 'NONE',  ( -0.5377323685532543474, 0.4294741335735779986, 0.1322818203437346463 ) ) ;
#13939=DIRECTION ( 'NONE',  ( 0.000000000000000000, 1.000000000000000000, 0.000000000000000000 ) ) ;
#13957=DIRECTION ( 'NONE',  ( 0.000000000000000000, 0.000000000000000000, 1.000000000000000000 ) ) ;
#13966=CARTESIAN_POINT ( 'NONE',  ( 0.6710470464557992676, -0.1526433524317950818, 0.3401591245381555551 ) ) ;
#13970=CYLINDRICAL_SURFACE ( 'NONE', #9550, 0.5322834645669292097 ) ;
#13981=AXIS2_PLACEMENT_3D ( 'NONE', #58, #21485, #21623 ) ;
#13988=CARTESIAN_POINT ( 'NONE',  ( -4.821444091131312140E-17, -0.3937007874015748254, 0.2362204724409449064 ) ) ;
#13992=DIRECTION ( 'NONE',  ( 0.000000000000000000, 0.000000000000000000, 1.000000000000000000 ) ) ;
#13995=CARTESIAN_POINT ( 'NONE',  ( -0.4681308612729627172, -0.1074986424507606841, 0.2362204724409447676 ) ) ;
#13999=VERTEX_POINT ( 'NONE', #14983 ) ;
#14035=CIRCLE ( 'NONE', #23059, 0.8031496062992127261 ) ;
#14066=EDGE_CURVE ( 'NONE', #26488, #25578, #12314, .T. ) ;
#14085=CARTESIAN_POINT ( 'NONE',  ( 0.5188388941967637669, -0.1188778293835250077, 0.3401591244667909186 ) ) ;
#14103=CARTESIAN_POINT ( 'NONE',  ( 0.6707652279343347956, -0.1538768215240155779, 0.3401574803149606252 ) ) ;
#14114=VERTEX_POINT ( 'NONE', #25979 ) ;
#14171=EDGE_CURVE ( 'NONE', #23254, #23881, #23455, .T. ) ;
#14175=DIRECTION ( 'NONE',  ( 0.000000000000000000, 0.000000000000000000, 1.000000000000000000 ) ) ;
#14179=DIRECTION ( 'NONE',  ( 0.000000000000000000, 0.000000000000000000, -1.000000000000000000 ) ) ;
#14191=CARTESIAN_POINT ( 'NONE',  ( 0.0006345105826660208141, 0.4803145415259080231, 0.2529987172466452994 ) ) ;
#14194=CIRCLE ( 'NONE', #19620, 0.1299232283464566984 ) ;
#14201=CARTESIAN_POINT ( 'NONE',  ( -0.0007595033562148819414, 0.6881885572739390167, 0.1322834645669291320 ) ) ;
#14214=FACE_OUTER_BOUND ( 'NONE', #22948, .T. ) ;
#14217=DIRECTION ( 'NONE',  ( 0.000000000000000000, 0.000000000000000000, 1.000000000000000000 ) ) ;
#14221=CARTESIAN_POINT ( 'NONE',  ( -0.5382052855068000241, 0.4288813374988110216, 0.1322810039474933141 ) ) ;
#14230=ORIENTED_EDGE ( 'NONE', *, *, #9868, .T. ) ;
#14233=DIRECTION ( 'NONE',  ( 0.4338837391175581759, -0.9009688679024190350, 0.000000000000000000 ) ) ;
#14243=DIRECTION ( 'NONE',  ( 1.000000000000000000, 0.000000000000000000, 0.000000000000000000 ) ) ;
#14247=ORIENTED_EDGE ( 'NONE', *, *, #24538, .F. ) ;
#14259=CIRCLE ( 'NONE', #4323, 0.5322834645669292097 ) ;
#14263=DIRECTION ( 'NONE',  ( 0.000000000000000000, 0.000000000000000000, 1.000000000000000000 ) ) ;
#14265=VERTEX_POINT ( 'NONE', #2771 ) ;
#14293=CARTESIAN_POINT ( 'NONE',  ( -0.2990496115119744003, -0.6198172806990825956, 0.3401591245381551110 ) ) ;
#14300=ORIENTED_EDGE ( 'NONE', *, *, #25752, .F. ) ;
#14314=DIRECTION ( 'NONE',  ( -1.000000000000000000, 0.000000000000000000, 0.000000000000000000 ) ) ;
#14340=EDGE_CURVE ( 'NONE', #11508, #23587, #7866, .T. ) ;
#14368=ORIENTED_EDGE ( 'NONE', *, *, #12729, .T. ) ;
#14373=EDGE_CURVE ( 'NONE', #16756, #21681, #5766, .T. ) ;
#14385=CARTESIAN_POINT ( 'NONE',  ( 0.5385210225480960844, 0.4284847435812472183, 0.3401574803149606252 ) ) ;
#14406=DIRECTION ( 'NONE',  ( 0.000000000000000000, 0.000000000000000000, -1.000000000000000000 ) ) ;
#14446=EDGE_CURVE ( 'NONE', #11422, #9678, #27790, .T. ) ;
#14447=CARTESIAN_POINT ( 'NONE',  ( -4.821444091131312140E-17, -0.3937007874015748254, 0.02362204724409448786 ) ) ;
#14464=TOROIDAL_SURFACE ( 'NONE', #26606, 0.6102362204724409711, 0.1299212598425196763 ) ;
#14471=ORIENTED_EDGE ( 'NONE', *, *, #901, .T. ) ;
#14475=CARTESIAN_POINT ( 'NONE',  ( -0.6996455634084097763, -0.1588938903144868908, 0.1601585119419891567 ) ) ;
#14476=DIRECTION ( 'NONE',  ( 1.000000000000000000, 0.000000000000000000, 0.000000000000000000 ) ) ;
#14486=AXIS2_PLACEMENT_3D ( 'NONE', #25169, #27301, #3696 ) ;
#14521=DIRECTION ( 'NONE',  ( 0.000000000000000000, 0.000000000000000000, 1.000000000000000000 ) ) ;
#14553=EDGE_CURVE ( 'NONE', #24778, #1564, #9540, .T. ) ;
#14565=FACE_OUTER_BOUND ( 'NONE', #7726, .T. ) ;
#14572=CARTESIAN_POINT ( 'NONE',  ( -0.4029514798600966063, 0.3205030004496360330, 0.3251195115602828478 ) ) ;
#14607=B_SPLINE_CURVE_WITH_KNOTS ( 'NONE', 3,
 ( #10317, #6109, #14746, #21210 ),
 .UNSPECIFIED., .F., .F.,
 ( 4, 4 ),
 ( 1.164573402063411978, 1.166266105206986037 ),
 .UNSPECIFIED. ) ;
#14614=( LENGTH_UNIT ( ) NAMED_UNIT ( * ) SI_UNIT ( $, .METRE. ) ) ;
#14625=EDGE_LOOP ( 'NONE', ( #23943, #15268 ) ) ;
#14626=TOROIDAL_SURFACE ( 'NONE', #13673, 0.6102362204724409711, 0.1299212598425196763 ) ;
#14627=CARTESIAN_POINT ( 'NONE',  ( -0.0006679551606482677165, 0.5322830454629158270, 0.1322834645669291320 ) ) ;
#14629=EDGE_CURVE ( 'NONE', #25578, #5717, #7873, .T. ) ;
#14634=CARTESIAN_POINT ( 'NONE',  ( 0.2104048168833876076, -0.4354435989199126888, 0.2715646632207475708 ) ) ;
#14684=VERTEX_POINT ( 'NONE', #24600 ) ;
#14707=ORIENTED_EDGE ( 'NONE', *, *, #5679, .F. ) ;
#14714=EDGE_CURVE ( 'NONE', #5717, #25431, #13260, .T. ) ;
#14732=CARTESIAN_POINT ( 'NONE',  ( 0.3062557396297003187, -0.6341756901040335181, 0.1443310008622352147 ) ) ;
#14736=DIRECTION ( 'NONE',  ( 0.000000000000000000, 0.000000000000000000, 1.000000000000000000 ) ) ;
#14743=EDGE_CURVE ( 'NONE', #12366, #1421, #8566, .T. ) ;
#14745=CIRCLE ( 'NONE', #21471, 0.8267716535433071723 ) ;
#14746=CARTESIAN_POINT ( 'NONE',  ( -0.0004447986960614961401, 0.5322833254990984031, 0.3401591244667909186 ) ) ;
#14777=CARTESIAN_POINT ( 'NONE',  ( 0.2089723435111816296, -0.4324731448915267173, 0.2529987172005040974 ) ) ;
#14840=ORIENTED_EDGE ( 'NONE', *, *, #14373, .T. ) ;
#14844=DIRECTION ( 'NONE',  ( 1.000000000000000000, 0.000000000000000000, 0.000000000000000000 ) ) ;
#14864=EDGE_LOOP ( 'NONE', ( #19181, #4689 ) ) ;
#14884=ORIENTED_EDGE ( 'NONE', *, *, #22420, .F. ) ;
#14886=DIRECTION ( 'NONE',  ( 0.000000000000000000, 0.000000000000000000, -1.000000000000000000 ) ) ;
#14903=CARTESIAN_POINT ( 'NONE',  ( -0.0002221395201540506592, 0.5322834645669292097, 0.1322810039474933141 ) ) ;
#14911=ADVANCED_FACE ( 'NONE', ( #22185 ), #11015, .F. ) ;
#14914=ORIENTED_EDGE ( 'NONE', *, *, #86, .F. ) ;
#14923=CARTESIAN_POINT ( 'NONE',  ( 0.000000000000000000, 0.000000000000000000, 0.02362204724409448786 ) ) ;
#14936=CIRCLE ( 'NONE', #5436, 0.4803149606299212393 ) ;
#14948=CARTESIAN_POINT ( 'NONE',  ( -0.6996455634166303117, -0.1588938903163411021, 0.3122824329290380674 ) ) ;
#14954=ORIENTED_EDGE ( 'NONE', *, *, #3378, .T. ) ;
#14957=EDGE_CURVE ( 'NONE', #26680, #26488, #3435, .T. ) ;
#14965=B_SPLINE_CURVE_WITH_KNOTS ( 'NONE', 3,
 ( #23782, #4280, #21931, #462, #26027, #4551, #12747, #19801 ),
 .UNSPECIFIED., .F., .F.,
 ( 4, 2, 2, 4 ),
 ( 0.000000000000000000, 0.1249999999999999445, 0.2500000000000000555, 0.5000000000000000000 ),
 .UNSPECIFIED. ) ;
#14969=CIRCLE ( 'NONE', #26640, 0.5322834645669292097 ) ;
#14976=AXIS2_PLACEMENT_3D ( 'NONE', #2533, #4254, #11156 ) ;
#14982=CARTESIAN_POINT ( 'NONE',  ( -0.6709908451338799651, -0.1528902114222696895, 0.1322810039474933141 ) ) ;
#14983=CARTESIAN_POINT ( 'NONE',  ( 0.6881889763779527325, 0.000000000000000000, 0.1322834645669291320 ) ) ;
#14986=SPHERICAL_SURFACE ( 'NONE', #21182, 0.1299232283464566984 ) ;
#14995=CARTESIAN_POINT ( 'NONE',  ( 0.3119936278817372344, -0.6460736482317533946, 0.1601585119437425875 ) ) ;
#14999=CARTESIAN_POINT ( 'NONE',  ( -0.3759206409296169671, 0.2989751379763689321, 0.2194422276316772835 ) ) ;
#15002=CARTESIAN_POINT ( 'NONE',  ( 0.2315507648392299000, -0.4792806379917101678, 0.3401574803149606252 ) ) ;
#15003=DIRECTION ( 'NONE',  ( 1.000000000000000000, 0.000000000000000000, 0.000000000000000000 ) ) ;
#15006=CARTESIAN_POINT ( 'NONE',  ( 0.000000000000000000, 0.3937007874015748254, 0.02362204724409448786 ) ) ;
#15008=SHAPE_REPRESENTATION ( 'Deep Groove Ball Bearing 20x42x12', ( #11588 ), #1261 ) ;
#15031=FACE_OUTER_BOUND ( 'NONE', #18070, .T. ) ;
#15054=CARTESIAN_POINT ( 'NONE',  ( -0.4173228346456693272, 5.110730736599190647E-17, 0.4724409448818898127 ) ) ;
#15056=ADVANCED_FACE ( 'NONE', ( #20629 ), #13292, .F. ) ;
#15058=DIRECTION ( 'NONE',  ( 1.000000000000000000, 0.000000000000000000, 0.000000000000000000 ) ) ;
#15059=CARTESIAN_POINT ( 'NONE',  ( 0.0006345105826664493992, 0.4803145415259079121, 0.2362204724409449896 ) ) ;
#15077=CARTESIAN_POINT ( 'NONE',  ( 0.000000000000000000, 0.000000000000000000, 0.4488188976377953110 ) ) ;
#15087=ORIENTED_EDGE ( 'NONE', *, *, #23719, .F. ) ;
#15088=B_SPLINE_CURVE_WITH_KNOTS ( 'NONE', 3,
 ( #18392, #14191, #20110, #3142, #5127, #22232, #18250, #768 ),
 .UNSPECIFIED., .F., .F.,
 ( 4, 2, 2, 4 ),
 ( 0.5000000000000000000, 0.7499999999999996669, 0.8749999999999997780, 1.000000000000000000 ),
 .UNSPECIFIED. ) ;
#15091=CYLINDRICAL_SURFACE ( 'NONE', #9049, 0.6881889763779527325 ) ;
#15095=EDGE_LOOP ( 'NONE', ( #11121, #22407, #27766, #10281, #793, #22438 ) ) ;
#15099=ORIENTED_EDGE ( 'NONE', *, *, #9420, .F. ) ;
#15113=AXIS2_PLACEMENT_3D ( 'NONE', #9144, #17763, #11410 ) ;
#15118=B_SPLINE_CURVE_WITH_KNOTS ( 'NONE', 3,
 ( #11234, #8840, #7009, #26347, #4477, #15765, #17464, #269 ),
 .UNSPECIFIED., .F., .F.,
 ( 4, 2, 2, 4 ),
 ( 0.000000000000000000, 0.1249999999999999722, 0.2499999999999999445, 0.5000000000000000000 ),
 .UNSPECIFIED. ) ;
#15121=EDGE_CURVE ( 'NONE', #15981, #14114, #16270, .T. ) ;
#15125=DIRECTION ( 'NONE',  ( -0.4338837391175582869, -0.9009688679024190350, 0.000000000000000000 ) ) ;
#15128=EDGE_CURVE ( 'NONE', #14684, #6454, #22759, .T. ) ;
#15141=CARTESIAN_POINT ( 'NONE',  ( 0.3882259019058474370, 0.3087756353523146702, 0.2989974301447032579 ) ) ;
#15175=CARTESIAN_POINT ( 'NONE',  ( -0.2983664441502653641, -0.6201464311010354002, 0.1322810039474933141 ) ) ;
#15181=DIRECTION ( 'NONE',  ( 0.000000000000000000, 0.000000000000000000, 1.000000000000000000 ) ) ;
#15210=CARTESIAN_POINT ( 'NONE',  ( -0.2078289949484350141, -0.4330237525397957477, 0.2362204724409447676 ) ) ;
#15253=ORIENTED_EDGE ( 'NONE', *, *, #7452, .T. ) ;
#15268=ORIENTED_EDGE ( 'NONE', *, *, #11269, .T. ) ;
#15276=CARTESIAN_POINT ( 'NONE',  ( -0.3924375359102375005, 0.3121297331111325124, 0.1643955689138890675 ) ) ;
#15277=ORIENTED_EDGE ( 'NONE', *, *, #2389, .F. ) ;
#15279=VERTEX_POINT ( 'NONE', #5945 ) ;
#15284=CARTESIAN_POINT ( 'NONE',  ( 0.4164331889188472857, 0.3315254675241992577, 0.1322818204150988386 ) ) ;
#15289=CIRCLE ( 'NONE', #21607, 0.6881889763779527325 ) ;
#15313=ADVANCED_FACE ( 'NONE', ( #23180, #4631 ), #682, .T. ) ;
#15317=AXIS2_PLACEMENT_3D ( 'NONE', #15598, #20091, #11070 ) ;
#15319=DIRECTION ( 'NONE',  ( 0.9009688679024190350, -0.4338837391175581204, 0.000000000000000000 ) ) ;
#15339=CARTESIAN_POINT ( 'NONE',  ( 0.2311492806687369950, -0.4794744477484330636, 0.3401599409343964431 ) ) ;
#15340=CARTESIAN_POINT ( 'NONE',  ( -0.5375739373539409893, 0.4296723508511055556, 0.1322834645669291320 ) ) ;
#15342=DIRECTION ( 'NONE',  ( 0.7818314824680296926, -0.6234898018587338164, 0.000000000000000000 ) ) ;
#15374=CARTESIAN_POINT ( 'NONE',  ( 0.4684132450478833976, -0.1062614382955264641, 0.2362204724409446843 ) ) ;
#15382=ORIENTED_EDGE ( 'NONE', *, *, #5207, .T. ) ;
#15398=EDGE_CURVE ( 'NONE', #19875, #27874, #7505, .T. ) ;
#15399=CIRCLE ( 'NONE', #10382, 0.6881889763779527325 ) ;
#15427=CARTESIAN_POINT ( 'NONE',  ( 0.2979095355690402069, -0.6203660015065080024, 0.1322834645669291320 ) ) ;
#15429=CARTESIAN_POINT ( 'NONE',  ( 0.6711032387266614441, -0.1523958994813204848, 0.1322834645669291320 ) ) ;
#15434=FACE_OUTER_BOUND ( 'NONE', #26257, .T. ) ;
#15452=CARTESIAN_POINT ( 'NONE',  ( 0.6711032387266614441, -0.1523958994813204848, 0.1322834645669291320 ) ) ;
#15453=DIRECTION ( 'NONE',  ( 0.000000000000000000, 0.000000000000000000, 1.000000000000000000 ) ) ;
#15463=CARTESIAN_POINT ( 'NONE',  ( -0.5510854067032040504, 0.4384931681280017091, 0.1443310008628239383 ) ) ;
#15491=EDGE_CURVE ( 'NONE', #13154, #21686, #19960, .T. ) ;
#15496=CIRCLE ( 'NONE', #6479, 0.4173228346456693272 ) ;
#15516=ADVANCED_FACE ( 'NONE', ( #2749 ), #1141, .F. ) ;
#15534=CARTESIAN_POINT ( 'NONE',  ( 0.0006345105826664493992, 0.4803145415259079121, 0.2362204724409449896 ) ) ;
#15538=DIRECTION ( 'NONE',  ( 0.000000000000000000, -1.000000000000000000, 0.000000000000000000 ) ) ;
#15542=VERTEX_POINT ( 'NONE', #8546 ) ;
#15561=DIRECTION ( 'NONE',  ( 0.000000000000000000, 0.000000000000000000, 1.000000000000000000 ) ) ;
#15562=CYLINDRICAL_SURFACE ( 'NONE', #5193, 0.3937007874015748254 ) ;
#15588=CARTESIAN_POINT ( 'NONE',  ( -8.427884271297532088E-17, -0.6881889763779527325, 0.1322834645669291320 ) ) ;
#15594=AXIS2_PLACEMENT_3D ( 'NONE', #13668, #9274, #26513 ) ;
#15598=CARTESIAN_POINT ( 'NONE',  ( 0.000000000000000000, 0.000000000000000000, 0.4724409448818898127 ) ) ;
#15602=AXIS2_PLACEMENT_3D ( 'NONE', #11048, #12882, #19671 ) ;
#15605=CARTESIAN_POINT ( 'NONE',  ( 0.2313498293151122209, -0.4793777142568558802, 0.1322818204150990051 ) ) ;
#15620=B_SPLINE_CURVE_WITH_KNOTS ( 'NONE', 3,
 ( #15821, #5513, #15961, #9169, #13692, #17787, #24849, #13840 ),
 .UNSPECIFIED., .F., .F.,
 ( 4, 2, 2, 4 ),
 ( 0.5000000000000000000, 0.7500000000000000000, 0.8750000000000000000, 1.000000000000000000 ),
 .UNSPECIFIED. ) ;
#15642=CARTESIAN_POINT ( 'NONE',  ( 0.4716287720755726887, -0.1069935333116613374, 0.2008762816168113419 ) ) ;
#15646=ORIENTED_EDGE ( 'NONE', *, *, #14066, .T. ) ;
#15652=ORIENTED_EDGE ( 'NONE', *, *, #19588, .F. ) ;
#15667=EDGE_LOOP ( 'NONE', ( #16679, #18810, #24723, #7185 ) ) ;
#15669=CARTESIAN_POINT ( 'NONE',  ( 0.3751294191746885609, 0.2999672986753447734, 0.2362204724409446843 ) ) ;
#15700=CARTESIAN_POINT ( 'NONE',  ( -0.4834654033798361228, -0.1110087727118397871, 0.1734435147621542217 ) ) ;
#15728=AXIS2_PLACEMENT_3D ( 'NONE', #5608, #24805, #10116 ) ;
#15730=EDGE_CURVE ( 'NONE', #27302, #16370, #11509, .T. ) ;
#15733=DIRECTION ( 'NONE',  ( 0.000000000000000000, 0.000000000000000000, 1.000000000000000000 ) ) ;
#15740=DIRECTION ( 'NONE',  ( 0.000000000000000000, 0.000000000000000000, 1.000000000000000000 ) ) ;
#15752=CARTESIAN_POINT ( 'NONE',  ( -0.2104048168850177758, -0.4354435989233408355, 0.2008762816475422042 ) ) ;
#15755=AXIS2_PLACEMENT_3D ( 'NONE', #11544, #13957, #2915 ) ;
#15757=ORIENTED_EDGE ( 'NONE', *, *, #20658, .F. ) ;
#15763=SHAPE_DEFINITION_REPRESENTATION ( #8681, #15008 ) ;
#15765=CARTESIAN_POINT ( 'NONE',  ( 0.3777066424217488949, 0.3020248451665031308, 0.2715646632922476544 ) ) ;
#15780=VERTEX_POINT ( 'NONE', #18600 ) ;
#15784=CARTESIAN_POINT ( 'NONE',  ( -0.4173228346456693272, 5.110730736599190647E-17, 0.4488188976377953110 ) ) ;
#15793=CARTESIAN_POINT ( 'NONE',  ( -0.2311492806687369950, -0.4794744477484330636, 0.1322810039474933141 ) ) ;
#15799=CARTESIAN_POINT ( 'NONE',  ( 0.000000000000000000, 0.6102362204724409711, -1.156053543307086666E-17 ) ) ;
#15806=CARTESIAN_POINT ( 'NONE',  ( 0.6864238947233102239, -0.1574599019769754027, 0.1443310008636487507 ) ) ;
#15807=ORIENTED_EDGE ( 'NONE', *, *, #19632, .T. ) ;
#15820=CARTESIAN_POINT ( 'NONE',  ( -0.3777066424189819971, 0.3020248451642900678, 0.2715646632795538085 ) ) ;
#15821=CARTESIAN_POINT ( 'NONE',  ( 0.4681308612729627727, -0.1074986424507606286, 0.2362204724409450174 ) ) ;
#15830=ORIENTED_EDGE ( 'NONE', *, *, #8188, .F. ) ;
#15831=DIRECTION ( 'NONE',  ( 0.000000000000000000, 0.000000000000000000, -1.000000000000000000 ) ) ;
#15843=TOROIDAL_SURFACE ( 'NONE', #3661, 0.6102362204724409711, 0.1299212598425196763 ) ;
#15844=CARTESIAN_POINT ( 'NONE',  ( 0.000000000000000000, 0.000000000000000000, 0.2362204724409449064 ) ) ;
#15851=DIRECTION ( 'NONE',  ( 0.000000000000000000, 1.000000000000000000, 0.000000000000000000 ) ) ;
#15861=CIRCLE ( 'NONE', #14976, 0.3937007874015748254 ) ;
#15862=EDGE_CURVE ( 'NONE', #18324, #3673, #25963, .T. ) ;
#15873=EDGE_CURVE ( 'NONE', #5084, #16925, #22379, .T. ) ;
#15896=SPHERICAL_SURFACE ( 'NONE', #2572, 0.1299232283464566984 ) ;
#15914=EDGE_CURVE ( 'NONE', #4492, #3371, #10929, .T. ) ;
#15920=CIRCLE ( 'NONE', #6453, 0.1299232283464566706 ) ;
#15925=EDGE_CURVE ( 'NONE', #13999, #11422, #26405, .T. ) ;
#15948=ADVANCED_FACE ( 'NONE', ( #26876 ), #7451, .F. ) ;
#15957=ORIENTED_EDGE ( 'NONE', *, *, #16581, .F. ) ;
#15959=DIRECTION ( 'NONE',  ( 1.000000000000000000, 0.000000000000000000, 0.000000000000000000 ) ) ;
#15961=CARTESIAN_POINT ( 'NONE',  ( 0.4713455951422338974, -0.1082342125229829866, 0.2715646632666751659 ) ) ;
#15973=CARTESIAN_POINT ( 'NONE',  ( 0.000000000000000000, 0.000000000000000000, 0.1322834645669291320 ) ) ;
#15978=CARTESIAN_POINT ( 'NONE',  ( -0.5949363243629232079, -0.1357903337134990229, 0.2362204724409449064 ) ) ;
#15979=CARTESIAN_POINT ( 'NONE',  ( -0.3119936278838151833, -0.6460736482360152078, 0.3122824329320355030 ) ) ;
#15981=VERTEX_POINT ( 'NONE', #7527 ) ;
#15983=CIRCLE ( 'NONE', #19607, 0.8267716535433071723 ) ;
#15985=EDGE_CURVE ( 'NONE', #15279, #21681, #26051, .T. ) ;
#15989=DIRECTION ( 'NONE',  ( 0.000000000000000000, 0.000000000000000000, -1.000000000000000000 ) ) ;
#16004=EDGE_CURVE ( 'NONE', #9013, #27602, #7188, .T. ) ;
#16007=DIRECTION ( 'NONE',  ( 0.000000000000000000, -1.000000000000000000, 0.000000000000000000 ) ) ;
#16024=AXIS2_PLACEMENT_3D ( 'NONE', #13180, #9077, #19697 ) ;
#16030=DIRECTION ( 'NONE',  ( 0.000000000000000000, 0.000000000000000000, 1.000000000000000000 ) ) ;
#16059=EDGE_LOOP ( 'NONE', ( #8202, #17312 ) ) ;
#16074=EDGE_CURVE ( 'NONE', #14684, #21440, #7023, .T. ) ;
#16079=ADVANCED_BREP_SHAPE_REPRESENTATION ( 'Deep Groove Ball Bearing 20x42x12', ( #12108, #11588 ), #1261 ) ;
#16105=LINE ( 'NONE', #13988, #6587 ) ;
#16113=CARTESIAN_POINT ( 'NONE',  ( 0.2078289949484098675, -0.4330237525398077381, 0.2529987172081292757 ) ) ;
#16118=ORIENTED_EDGE ( 'NONE', *, *, #5679, .T. ) ;
#16152=CARTESIAN_POINT ( 'NONE',  ( 0.000000000000000000, 0.000000000000000000, 0.2362204724409449064 ) ) ;
#16157=LENGTH_MEASURE_WITH_UNIT ( LENGTH_MEASURE( 0.02539999999999999897 ), #19032 ) ;
#16182=ADVANCED_FACE ( 'NONE', ( #6959, #87 ), #2556, .T. ) ;
#16183=CIRCLE ( 'NONE', #26545, 0.02362204724409448092 ) ;
#16193=CYLINDRICAL_SURFACE ( 'NONE', #8685, 0.5322834645669292097 ) ;
#16198=DIRECTION ( 'NONE',  ( 0.000000000000000000, 0.000000000000000000, 1.000000000000000000 ) ) ;
#16202=ADVANCED_FACE ( 'NONE', ( #10915 ), #13767, .F. ) ;
#16212=EDGE_LOOP ( 'NONE', ( #18481, #15807, #428, #9788, #16754 ) ) ;
#16224=ORIENTED_EDGE ( 'NONE', *, *, #17233, .T. ) ;
#16255=CARTESIAN_POINT ( 'NONE',  ( -0.4021324607151492980, 0.3215300179757064614, 0.1473214333199995008 ) ) ;
#16267=DIRECTION ( 'NONE',  ( 1.000000000000000000, 0.000000000000000000, 0.000000000000000000 ) ) ;
#16270=B_SPLINE_CURVE_WITH_KNOTS ( 'NONE', 3,
 ( #3514, #24996, #16255, #3226, #24574, #11865, #18486, #20486 ),
 .UNSPECIFIED., .F., .F.,
 ( 4, 2, 2, 4 ),
 ( 0.000000000000000000, 0.1250000000000000000, 0.2499999999999998335, 0.5000000000000000000 ),
 .UNSPECIFIED. ) ;
#16279=ADVANCED_FACE ( 'NONE', ( #20498 ), #14464, .F. ) ;
#16286=CARTESIAN_POINT ( 'NONE',  ( -0.4158785340170984557, 0.3322209827720822850, 0.3401591244667909186 ) ) ;
#16292=CARTESIAN_POINT ( 'NONE',  ( 0.3218523081053298873, -0.6665164569875627887, 0.2562996995945706069 ) ) ;
#16302=DIRECTION ( 'NONE',  ( 0.000000000000000000, 1.000000000000000000, 0.000000000000000000 ) ) ;
#16308=ADVANCED_FACE ( 'NONE', ( #13714 ), #5008, .T. ) ;
#16320=AXIS2_PLACEMENT_3D ( 'NONE', #11347, #22505, #1041 ) ;
#16327=ORIENTED_EDGE ( 'NONE', *, *, #21317, .F. ) ;
#16331=CARTESIAN_POINT ( 'NONE',  ( -0.5375739373539409893, 0.4296723508511055556, 0.1322834645669291320 ) ) ;
#16352=AXIS2_PLACEMENT_3D ( 'NONE', #7151, #2889, #11115 ) ;
#16365=ORIENTED_EDGE ( 'NONE', *, *, #24251, .T. ) ;
#16370=VERTEX_POINT ( 'NONE', #26849 ) ;
#16390=ORIENTED_EDGE ( 'NONE', *, *, #15914, .T. ) ;
#16391=VERTEX_POINT ( 'NONE', #20213 ) ;
#16416=EDGE_LOOP ( 'NONE', ( #6168, #19443, #17867, #6339, #20325 ) ) ;
#16417=CARTESIAN_POINT ( 'NONE',  ( -0.4162944719209866196, 0.3316996361851582975, 0.3401599409343964431 ) ) ;
#16422=DIRECTION ( 'NONE',  ( 1.224646799147353207E-16, 1.000000000000000000, -0.000000000000000000 ) ) ;
#16431=CARTESIAN_POINT ( 'NONE',  ( -0.0007756954652713807415, 0.7174612052785541705, 0.3122824329337317018 ) ) ;
#16447=CARTESIAN_POINT ( 'NONE',  ( -0.0006679551606482677165, 0.5322830454629158270, 0.1322834645669291320 ) ) ;
#16449=ORIENTED_EDGE ( 'NONE', *, *, #15730, .T. ) ;
#16478=DIRECTION ( 'NONE',  ( -0.7818314824680295816, 0.6234898018587339275, 0.000000000000000000 ) ) ;
#16483=AXIS2_PLACEMENT_3D ( 'NONE', #21956, #15342, #17427 ) ;
#16486=EDGE_CURVE ( 'NONE', #11391, #22315, #22342, .T. ) ;
#16487=CARTESIAN_POINT ( 'NONE',  ( 0.4771018889076559244, 0.3804760601893846794, 0.3661437007874016047 ) ) ;
#16498=CARTESIAN_POINT ( 'NONE',  ( 0.6102362204724409711, 0.000000000000000000, 0.2362204724409449064 ) ) ;
#16511=VERTEX_POINT ( 'NONE', #8760 ) ;
#16531=ORIENTED_EDGE ( 'NONE', *, *, #14629, .T. ) ;
#16535=CARTESIAN_POINT ( 'NONE',  ( -0.2104048168856049172, -0.4354435989245551419, 0.2715646632391802151 ) ) ;
#16581=EDGE_CURVE ( 'NONE', #21208, #19384, #6328, .T. ) ;
#16591=ORIENTED_EDGE ( 'NONE', *, *, #10114, .T. ) ;
#16609=VERTEX_POINT ( 'NONE', #23617 ) ;
#16642=AXIS2_PLACEMENT_3D ( 'NONE', #22045, #22321, #11308 ) ;
#16648=B_SPLINE_CURVE_WITH_KNOTS ( 'NONE', 3,
 ( #5598, #9031, #18289, #27214 ),
 .UNSPECIFIED., .F., .F.,
 ( 4, 4 ),
 ( 1.162880698919837918, 1.164573402063411978 ),
 .UNSPECIFIED. ) ;
#16657=VERTEX_POINT ( 'NONE', #4114 ) ;
#16658=EDGE_CURVE ( 'NONE', #6454, #20576, #6319, .T. ) ;
#16659=CARTESIAN_POINT ( 'NONE',  ( 0.000000000000000000, 0.000000000000000000, 0.2362204724409449064 ) ) ;
#16663=EDGE_CURVE ( 'NONE', #21686, #23531, #25025, .T. ) ;
#16679=ORIENTED_EDGE ( 'NONE', *, *, #12729, .F. ) ;
#16693=CARTESIAN_POINT ( 'NONE',  ( -0.2274877609461333494, -0.4708572476091899550, 0.3331434174514416036 ) ) ;
#16715=ORIENTED_EDGE ( 'NONE', *, *, #27081, .T. ) ;
#16724=AXIS2_PLACEMENT_3D ( 'NONE', #20288, #16198, #22262 ) ;
#16754=ORIENTED_EDGE ( 'NONE', *, *, #21609, .T. ) ;
#16755=ORIENTED_EDGE ( 'NONE', *, *, #17223, .T. ) ;
#16756=VERTEX_POINT ( 'NONE', #19911 ) ;
#16771=CARTESIAN_POINT ( 'NONE',  ( 0.2313498293151122209, -0.4793777142568558802, 0.3401591244667909186 ) ) ;
#16772=DIRECTION ( 'NONE',  ( 0.000000000000000000, 1.000000000000000000, 0.000000000000000000 ) ) ;
#16789=ORIENTED_EDGE ( 'NONE', *, *, #27081, .F. ) ;
#16823=CARTESIAN_POINT ( 'NONE',  ( 0.2992781133268291316, -0.6197069291944922176, 0.1322834645669291320 ) ) ;
#16824=EDGE_CURVE ( 'NONE', #15542, #27306, #12230, .T. ) ;
#16837=CARTESIAN_POINT ( 'NONE',  ( -0.2089723435111595362, -0.4324731448915372645, 0.2529987172187860844 ) ) ;
#16842=EDGE_LOOP ( 'NONE', ( #24381, #1281 ) ) ;
#16865=CARTESIAN_POINT ( 'NONE',  ( -7.279147705782180972E-18, 0.5322834645669292097, 0.1322810039474933141 ) ) ;
#16866=CARTESIAN_POINT ( 'NONE',  ( 0.000000000000000000, 0.000000000000000000, 0.4488188976377953110 ) ) ;
#16891=ORIENTED_EDGE ( 'NONE', *, *, #10960, .T. ) ;
#16909=LINE ( 'NONE', #21426, #22095 ) ;
#16922=VERTEX_POINT ( 'NONE', #24765 ) ;
#16925=VERTEX_POINT ( 'NONE', #17965 ) ;
#16937=ORIENTED_EDGE ( 'NONE', *, *, #14171, .T. ) ;
#16974=DIRECTION ( 'NONE',  ( 0.000000000000000000, 0.000000000000000000, 1.000000000000000000 ) ) ;
#16978=DIRECTION ( 'NONE',  ( 0.000000000000000000, 0.000000000000000000, 1.000000000000000000 ) ) ;
#16980=CARTESIAN_POINT ( 'NONE',  ( 0.3937007874015748254, 0.000000000000000000, 0.4488188976377953110 ) ) ;
#17014=VERTEX_POINT ( 'NONE', #22518 ) ;
#17029=CARTESIAN_POINT ( 'NONE',  ( -0.6710470464557992676, -0.1526433524317946933, 0.3401591245381555551 ) ) ;
#17047=DIRECTION ( 'NONE',  ( 0.000000000000000000, 0.000000000000000000, 1.000000000000000000 ) ) ;
#17055=ORIENTED_EDGE ( 'NONE', *, *, #7697, .F. ) ;
#17082=VERTEX_POINT ( 'NONE', #3864 ) ;
#17083=CARTESIAN_POINT ( 'NONE',  ( 0.5322834645669292097, 0.000000000000000000, 0.3401574803149606252 ) ) ;
#17088=FACE_OUTER_BOUND ( 'NONE', #14625, .T. ) ;
#17090=CARTESIAN_POINT ( 'NONE',  ( -0.5190862322091315262, -0.1177929122753175184, 0.1322834645669291320 ) ) ;
#17099=DIRECTION ( 'NONE',  ( 0.000000000000000000, 1.000000000000000000, 0.000000000000000000 ) ) ;
#17100=CARTESIAN_POINT ( 'NONE',  ( 0.0007856387884297636034, 0.7354206117094393980, 0.1960773254400930421 ) ) ;
#17114=CARTESIAN_POINT ( 'NONE',  ( -0.5190862322091315262, -0.1177929122753175184, 0.1322834645669291320 ) ) ;
#17144=AXIS2_PLACEMENT_3D ( 'NONE', #21319, #12559, #21176 ) ;
#17146=CARTESIAN_POINT ( 'NONE',  ( -0.2303471512294322787, -0.4798602677570401598, 0.1322834645669291320 ) ) ;
#17162=AXIS2_PLACEMENT_3D ( 'NONE', #22553, #24520, #3035 ) ;
#17172=MECHANICAL_DESIGN_GEOMETRIC_PRESENTATION_REPRESENTATION('',(#2279),#956);
#17217=DIRECTION ( 'NONE',  ( 0.4338837391175581759, -0.9009688679024190350, 0.000000000000000000 ) ) ;
#17220=DIRECTION ( 'NONE',  ( 0.000000000000000000, 0.000000000000000000, 1.000000000000000000 ) ) ;
#17223=EDGE_CURVE ( 'NONE', #16511, #21309, #27095, .T. ) ;
#17233=EDGE_CURVE ( 'NONE', #9309, #22865, #5421, .T. ) ;
#17250=CARTESIAN_POINT ( 'NONE',  ( -0.5021077788545322829, -0.1139291307079571824, 0.1473214333301098022 ) ) ;
#17257=TOROIDAL_SURFACE ( 'NONE', #24445, 0.6102362204724409711, 0.1299212598425196763 ) ;
#17274=CARTESIAN_POINT ( 'NONE',  ( 0.4681308612729627727, -0.1074986424507606286, 0.2362204724409450174 ) ) ;
#17277=EDGE_LOOP ( 'NONE', ( #23753, #942 ) ) ;
#17291=EDGE_CURVE ( 'NONE', #21258, #13825, #8870, .T. ) ;
#17294=CIRCLE ( 'NONE', #20909, 0.5322834645669292097 ) ;
#17296=AXIS2_PLACEMENT_3D ( 'NONE', #15844, #24319, #9194 ) ;
#17297=CARTESIAN_POINT ( 'NONE',  ( 0.000000000000000000, 0.000000000000000000, 0.1322834645669291320 ) ) ;
#17299=DIRECTION ( 'NONE',  ( 0.000000000000000000, 0.000000000000000000, 1.000000000000000000 ) ) ;
#17303=ORIENTED_EDGE ( 'NONE', *, *, #11181, .T. ) ;
#17309=AXIS2_PLACEMENT_3D ( 'NONE', #39, #4232, #2511 ) ;
#17312=ORIENTED_EDGE ( 'NONE', *, *, #15862, .T. ) ;
#17315=DIRECTION ( 'NONE',  ( 0.000000000000000000, 1.000000000000000000, 0.000000000000000000 ) ) ;
#17316=DIRECTION ( 'NONE',  ( 0.000000000000000000, 0.000000000000000000, -1.000000000000000000 ) ) ;
#17366=CARTESIAN_POINT ( 'NONE',  ( -0.5188388941967637669, -0.1188778293835246053, 0.1322818204150990051 ) ) ;
#17377=CARTESIAN_POINT ( 'NONE',  ( 0.0007683673430012761965, 0.7042519390037932370, 0.3281099440175705984 ) ) ;
#17384=CARTESIAN_POINT ( 'NONE',  ( 0.4158785340170984557, 0.3322209827720822850, 0.1322818204150988386 ) ) ;
#17406=CARTESIAN_POINT ( 'NONE',  ( -0.2647715730835492609, -0.5498038367121063086, 0.2362204724409449064 ) ) ;
#17407=ADVANCED_FACE ( 'NONE', ( #5392 ), #21092, .T. ) ;
#17410=PRODUCT_DEFINITION ( 'UNKNOWN', '', #10661, #9664 ) ;
#17423=CARTESIAN_POINT ( 'NONE',  ( -0.5375739373539409893, 0.4296723508511047229, 0.3401574803149606252 ) ) ;
#17426=ORIENTED_EDGE ( 'NONE', *, *, #5572, .F. ) ;
#17427=DIRECTION ( 'NONE',  ( 0.6234898018587334834, 0.7818314824680296926, 0.000000000000000000 ) ) ;
#17435=DIRECTION ( 'NONE',  ( 1.000000000000000000, 0.000000000000000000, 0.000000000000000000 ) ) ;
#17454=EDGE_CURVE ( 'NONE', #1755, #23254, #14607, .T. ) ;
#17464=CARTESIAN_POINT ( 'NONE',  ( 0.3751294191746887274, 0.2999672986753446624, 0.2529987172518466387 ) ) ;
#17476=ORIENTED_EDGE ( 'NONE', *, *, #19683, .T. ) ;
#17480=VERTEX_POINT ( 'NONE', #27572 ) ;
#17481=EDGE_LOOP ( 'NONE', ( #23966, #3456, #15382, #27109, #12488 ) ) ;
#17490=AXIS2_PLACEMENT_3D ( 'NONE', #4840, #1183, #17694 ) ;
#17500=EDGE_LOOP ( 'NONE', ( #2280, #21524, #8970, #17664, #5098, #10613 ) ) ;
#17510=CARTESIAN_POINT ( 'NONE',  ( 0.7214243740400071436, -0.1654689342656250894, 0.2161412452787339344 ) ) ;
#17512=AXIS2_PLACEMENT_3D ( 'NONE', #26160, #19672, #6537 ) ;
#17522=CIRCLE ( 'NONE', #5337, 0.1299232283464567539 ) ;
#17525=CARTESIAN_POINT ( 'NONE',  ( -0.3874223757830720927, 0.3097832252370624206, 0.2989974301407470891 ) ) ;
#17530=EDGE_CURVE ( 'NONE', #23783, #17886, #9833, .T. ) ;
#17536=CARTESIAN_POINT ( 'NONE',  ( 0.000000000000000000, 0.000000000000000000, 0.2362204724409449064 ) ) ;
#17538=CARTESIAN_POINT ( 'NONE',  ( -0.4684132450478833976, -0.1062614382955279213, 0.2529987172372142878 ) ) ;
#17554=CARTESIAN_POINT ( 'NONE',  ( 0.5190862322091315262, -0.1177929122753177127, 0.3401574803149606252 ) ) ;
#17556=CARTESIAN_POINT ( 'NONE',  ( 5.827097576719993621E-17, 0.6881889763779529545, 0.3401599409343964431 ) ) ;
#17574=EDGE_CURVE ( 'NONE', #18836, #13154, #18921, .T. ) ;
#17603=VECTOR ( 'NONE', #3848, 39.37007874015748143 ) ;
#17605=CARTESIAN_POINT ( 'NONE',  ( 0.5385210225480960844, 0.4284847435812472183, 0.1322834645669291320 ) ) ;
#17664=ORIENTED_EDGE ( 'NONE', *, *, #10960, .F. ) ;
#17694=DIRECTION ( 'NONE',  ( 0.000000000000000000, -1.000000000000000000, 0.000000000000000000 ) ) ;
#17701=LINE ( 'NONE', #7245, #20416 ) ;
#17703=AXIS2_PLACEMENT_3D ( 'NONE', #20104, #26326, #626 ) ;
#17725=CARTESIAN_POINT ( 'NONE',  ( 0.5099673189337476931, -0.1157175986333582596, 0.3331434174568621565 ) ) ;
#17748=CARTESIAN_POINT ( 'NONE',  ( -0.3183792087434620388, -0.6629319518604491757, 0.2763636194374882171 ) ) ;
#17763=DIRECTION ( 'NONE',  ( -0.9749279121818236193, -0.2225209339563142819, 0.000000000000000000 ) ) ;
#17776=CARTESIAN_POINT ( 'NONE',  ( 0.5375739373539409893, 0.4296723508511047229, 0.3401574803149606252 ) ) ;
#17781=DIRECTION ( 'NONE',  ( 0.000000000000000000, 1.000000000000000000, 0.000000000000000000 ) ) ;
#17787=CARTESIAN_POINT ( 'NONE',  ( 0.5018154743078061530, -0.1152098006148895432, 0.3251195115541528069 ) ) ;
#17802=DIRECTION ( 'NONE',  ( -0.4338837391175582314, -0.9009688679024192570, 0.000000000000000000 ) ) ;
#17803=ORIENTED_EDGE ( 'NONE', *, *, #27799, .T. ) ;
#17810=CARTESIAN_POINT ( 'NONE',  ( 0.8031496062992127261, 0.000000000000000000, 0.02362204724409448786 ) ) ;
#17813=CARTESIAN_POINT ( 'NONE',  ( 7.955503286468943460E-18, 0.6102362204724409711, 0.1062972440944881941 ) ) ;
#17827=VECTOR ( 'NONE', #22472, 39.37007874015748143 ) ;
#17836=VERTEX_POINT ( 'NONE', #12129 ) ;
#17847=DIRECTION ( 'NONE',  ( -0.9749279121818235083, 0.2225209339563148925, 0.000000000000000000 ) ) ;
#17853=ORIENTED_EDGE ( 'NONE', *, *, #1539, .F. ) ;
#17866=ORIENTED_EDGE ( 'NONE', *, *, #8957, .F. ) ;
#17867=ORIENTED_EDGE ( 'NONE', *, *, #20791, .T. ) ;
#17886=VERTEX_POINT ( 'NONE', #21177 ) ;
#17900=ORIENTED_EDGE ( 'NONE', *, *, #2014, .F. ) ;
#17915=ORIENTED_EDGE ( 'NONE', *, *, #15128, .F. ) ;
#17922=ADVANCED_FACE ( 'NONE', ( #27257, #7906 ), #1542, .T. ) ;
#17932=CIRCLE ( 'NONE', #18865, 0.6881889763779527325 ) ;
#17940=DIRECTION ( 'NONE',  ( 0.000000000000000000, 1.000000000000000000, 0.000000000000000000 ) ) ;
#17946=AXIS2_PLACEMENT_3D ( 'NONE', #8051, #17217, #12834 ) ;
#17951=CARTESIAN_POINT ( 'NONE',  ( 0.2181459867426673305, -0.4514914376958676923, 0.1643955689704863221 ) ) ;
#17955=CIRCLE ( 'NONE', #1321, 0.6881889763779527325 ) ;
#17965=CARTESIAN_POINT ( 'NONE',  ( 0.2315507648392299000, -0.4792806379917101678, 0.1322834645669291320 ) ) ;
#17986=FACE_OUTER_BOUND ( 'NONE', #23376, .T. ) ;
#17998=ORIENTED_EDGE ( 'NONE', *, *, #8243, .T. ) ;
#18003=CARTESIAN_POINT ( 'NONE',  ( 0.000000000000000000, 0.000000000000000000, 0.1322834645669291320 ) ) ;
#18006=VECTOR ( 'NONE', #24282, 39.37007874015748143 ) ;
#18008=DIRECTION ( 'NONE',  ( 0.000000000000000000, 0.000000000000000000, 1.000000000000000000 ) ) ;
#18009=CARTESIAN_POINT ( 'NONE',  ( 0.5188885761056504231, -0.1186607836835330693, 0.3401599409343964431 ) ) ;
#18026=AXIS2_PLACEMENT_3D ( 'NONE', #30, #23981, #4619 ) ;
#18037=CARTESIAN_POINT ( 'NONE',  ( -0.0007595033562148819414, 0.6881885572739390167, 0.1322834645669291320 ) ) ;
#18057=VERTEX_POINT ( 'NONE', #2231 ) ;
#18058=CARTESIAN_POINT ( 'NONE',  ( 0.000000000000000000, 0.000000000000000000, 0.4488188976377953110 ) ) ;
#18065=EDGE_CURVE ( 'NONE', #21624, #11391, #13863, .T. ) ;
#18070=EDGE_LOOP ( 'NONE', ( #26901, #26566, #24801, #26737, #16755, #17426, #6754, #5166, #1837, #20841, #9524, #16390 ) ) ;
#18075=FACE_BOUND ( 'NONE', #2662, .T. ) ;
#18077=CARTESIAN_POINT ( 'NONE',  ( 0.000000000000000000, 0.000000000000000000, 0.1322834645669291320 ) ) ;
#18078=CARTESIAN_POINT ( 'NONE',  ( 0.5378903297326614874, 0.4292762795476984805, 0.1322810039474933141 ) ) ;
#18083=CARTESIAN_POINT ( 'NONE',  ( 0.2274877609429545866, -0.4708572476026047227, 0.1392975274359326554 ) ) ;
#18092=ORIENTED_EDGE ( 'NONE', *, *, #1474, .F. ) ;
#18104=EDGE_CURVE ( 'NONE', #5702, #25047, #21605, .T. ) ;
#18146=CARTESIAN_POINT ( 'NONE',  ( -0.8267716535433071723, 1.012503259137575512E-16, 0.4488188976377953110 ) ) ;
#18161=CYLINDRICAL_SURFACE ( 'NONE', #12855, 0.6881889763779527325 ) ;
#18165=PLANE ( 'NONE',  #22801 ) ;
#18167=CARTESIAN_POINT ( 'NONE',  ( 0.4165721057576322606, 0.3313508221749649763, 0.1322834645669291320 ) ) ;
#18172=ORIENTED_EDGE ( 'NONE', *, *, #1366, .T. ) ;
#18189=EDGE_CURVE ( 'NONE', #4754, #27858, #17522, .T. ) ;
#18191=DIRECTION ( 'NONE',  ( 0.000000000000000000, 0.000000000000000000, 1.000000000000000000 ) ) ;
#18192=AXIS2_PLACEMENT_3D ( 'NONE', #17536, #13150, #21777 ) ;
#18198=CARTESIAN_POINT ( 'NONE',  ( 0.000000000000000000, 0.000000000000000000, 0.3401574803149606252 ) ) ;
#18203=ORIENTED_EDGE ( 'NONE', *, *, #4865, .F. ) ;
#18214=ORIENTED_EDGE ( 'NONE', *, *, #9320, .F. ) ;
#18221=CARTESIAN_POINT ( 'NONE',  ( -0.2303471512294322787, -0.4798602677570401598, 0.3401574803149606252 ) ) ;
#18231=CARTESIAN_POINT ( 'NONE',  ( -0.4164331889188472857, 0.3315254675241992577, 0.3401591244667909186 ) ) ;
#18238=CARTESIAN_POINT ( 'NONE',  ( 0.2315507648392299000, -0.4792806379917101678, 0.1322834645669291320 ) ) ;
#18239=ORIENTED_EDGE ( 'NONE', *, *, #21609, .F. ) ;
#18240=EDGE_CURVE ( 'NONE', #9314, #10270, #12113, .T. ) ;
#18250=CARTESIAN_POINT ( 'NONE',  ( 0.0006620872580293073444, 0.5229309616560341434, 0.3331434174597993625 ) ) ;
#18258=CARTESIAN_POINT ( 'NONE',  ( -0.2089723435111590921, -0.4324731448915377641, 0.2362204724409450174 ) ) ;
#18272=EDGE_CURVE ( 'NONE', #17082, #4219, #19013, .T. ) ;
#18286=AXIS2_PLACEMENT_3D ( 'NONE', #9734, #5509, #15959 ) ;
#18289=CARTESIAN_POINT ( 'NONE',  ( 0.0002221395201540944610, 0.5322834645669292097, 0.3401599409343964431 ) ) ;
#18293=EDGE_CURVE ( 'NONE', #25047, #11425, #23433, .T. ) ;
#18319=EDGE_CURVE ( 'NONE', #6332, #19539, #8094, .T. ) ;
#18324=VERTEX_POINT ( 'NONE', #17813 ) ;
#18328=B_SPLINE_CURVE_WITH_KNOTS ( 'NONE', 3,
 ( #15669, #2657, #22152, #24001, #4637, #2245, #19900, #25988 ),
 .UNSPECIFIED., .F., .F.,
 ( 4, 2, 2, 4 ),
 ( 0.5000000000000000000, 0.7499999999999998890, 0.8750000000000000000, 1.000000000000000000 ),
 .UNSPECIFIED. ) ;
#18344=DIRECTION ( 'NONE',  ( 0.000000000000000000, 1.000000000000000000, 0.000000000000000000 ) ) ;
#18362=CIRCLE ( 'NONE', #20177, 0.1299232283464566984 ) ;
#18388=ORIENTED_EDGE ( 'NONE', *, *, #12754, .T. ) ;
#18392=CARTESIAN_POINT ( 'NONE',  ( 0.0006345105826664493992, 0.4803145415259079121, 0.2362204724409449896 ) ) ;
#18401=DIRECTION ( 'NONE',  ( 0.2225209339563138933, -0.9749279121818237304, 0.000000000000000000 ) ) ;
#18423=AXIS2_PLACEMENT_3D ( 'NONE', #22063, #8696, #17315 ) ;
#18479=CARTESIAN_POINT ( 'NONE',  ( -0.4165721057576322606, 0.3313508221749649763, 0.3401574803149606252 ) ) ;
#18481=ORIENTED_EDGE ( 'NONE', *, *, #18104, .F. ) ;
#18486=CARTESIAN_POINT ( 'NONE',  ( -0.3751294191746890050, 0.2999672986753444404, 0.2194422276354875134 ) ) ;
#18502=EDGE_CURVE ( 'NONE', #27673, #22433, #13046, .T. ) ;
#18507=ORIENTED_EDGE ( 'NONE', *, *, #4066, .F. ) ;
#18540=DIRECTION ( 'NONE',  ( -1.000000000000000000, 1.224646799147353454E-16, 0.000000000000000000 ) ) ;
#18555=DIRECTION ( 'NONE',  ( 0.000000000000000000, -1.000000000000000000, 0.000000000000000000 ) ) ;
#18560=CARTESIAN_POINT ( 'NONE',  ( 0.2228021814271965440, -0.4641672719422391125, 0.1473214333490711070 ) ) ;
#18573=FACE_OUTER_BOUND ( 'NONE', #23413, .T. ) ;
#18575=DIRECTION ( 'NONE',  ( -0.6234898018587338164, -0.7818314824680293595, 0.000000000000000000 ) ) ;
#18582=CARTESIAN_POINT ( 'NONE',  ( 0.5190862322091315262, -0.1177929122753177127, 0.3401574803149606252 ) ) ;
#18587=AXIS2_PLACEMENT_3D ( 'NONE', #10599, #19223, #27855 ) ;
#18595=EDGE_LOOP ( 'NONE', ( #18964, #13401, #3063, #25367, #338 ) ) ;
#18600=CARTESIAN_POINT ( 'NONE',  ( -6.518592411209533944E-17, -0.5322834645669292097, 0.1322834645669291320 ) ) ;
#18613=TOROIDAL_SURFACE ( 'NONE', #24449, 0.6102362204724409711, 0.1299212598425196763 ) ;
#18632=CIRCLE ( 'NONE', #22250, 0.1299232283464567261 ) ;
#18634=ORIENTED_EDGE ( 'NONE', *, *, #17223, .F. ) ;
#18647=AXIS2_PLACEMENT_3D ( 'NONE', #5107, #24599, #13731 ) ;
#18663=TOROIDAL_SURFACE ( 'NONE', #18192, 0.6102362204724409711, 0.1299212598425196763 ) ;
#18668=CYLINDRICAL_SURFACE ( 'NONE', #25379, 0.5322834645669292097 ) ;
#18669=EDGE_CURVE ( 'NONE', #17886, #16657, #3564, .T. ) ;
#18672=ORIENTED_EDGE ( 'NONE', *, *, #18669, .T. ) ;
#18682=CARTESIAN_POINT ( 'NONE',  ( 0.000000000000000000, 0.000000000000000000, 0.4488188976377953110 ) ) ;
#18700=CARTESIAN_POINT ( 'NONE',  ( 0.5375739373539409893, 0.4296723508511047229, 0.3401574803149606252 ) ) ;
#18748=ORIENTED_EDGE ( 'NONE', *, *, #23502, .T. ) ;
#18752=EDGE_CURVE ( 'NONE', #11291, #26680, #12608, .T. ) ;
#18792=ORIENTED_EDGE ( 'NONE', *, *, #22959, .F. ) ;
#18810=ORIENTED_EDGE ( 'NONE', *, *, #26814, .F. ) ;
#18824=ORIENTED_EDGE ( 'NONE', *, *, #15925, .F. ) ;
#18836=VERTEX_POINT ( 'NONE', #910 ) ;
#18845=DIRECTION ( 'NONE',  ( 0.000000000000000000, 0.000000000000000000, 1.000000000000000000 ) ) ;
#18865=AXIS2_PLACEMENT_3D ( 'NONE', #6969, #15181, #21667 ) ;
#18880=VECTOR ( 'NONE', #1236, 39.37007874015748143 ) ;
#18906=CARTESIAN_POINT ( 'NONE',  ( -0.3759206409296168561, 0.2989751379763687655, 0.2362204724409447676 ) ) ;
#18921=B_SPLINE_CURVE_WITH_KNOTS ( 'NONE', 3,
 ( #64, #17384, #8897, #12861, #15284, #26139 ),
 .UNSPECIFIED., .F., .F.,
 ( 4, 2, 4 ),
 ( 0.3864984308775630262, 0.3881911340211369743, 0.3898838371647120327 ),
 .UNSPECIFIED. ) ;
#18937=ADVANCED_FACE ( 'NONE', ( #9834, #18573 ), #809, .T. ) ;
#18941=CARTESIAN_POINT ( 'NONE',  ( -7.279147705782180972E-18, 0.5322834645669292097, 0.1322810039474933141 ) ) ;
#18950=AXIS2_PLACEMENT_3D ( 'NONE', #16659, #6216, #14844 ) ;
#18964=ORIENTED_EDGE ( 'NONE', *, *, #12829, .T. ) ;
#18975=DIRECTION ( 'NONE',  ( 0.000000000000000000, 1.000000000000000000, 0.000000000000000000 ) ) ;
#18997=DIRECTION ( 'NONE',  ( 0.000000000000000000, -1.000000000000000000, 0.000000000000000000 ) ) ;
#19013=LINE ( 'NONE', #5898, #18880 ) ;
#19032=( LENGTH_UNIT ( ) NAMED_UNIT ( * ) SI_UNIT ( $, .METRE. ) ) ;
#19081=ORIENTED_EDGE ( 'NONE', *, *, #1720, .T. ) ;
#19096=LENGTH_MEASURE_WITH_UNIT ( LENGTH_MEASURE( 0.02539999999999999897 ), #14614 ) ;
#19110=FACE_OUTER_BOUND ( 'NONE', #20138, .T. ) ;
#19147=CARTESIAN_POINT ( 'NONE',  ( 0.000000000000000000, 0.000000000000000000, 0.4724409448818898127 ) ) ;
#19167=ADVANCED_FACE ( 'NONE', ( #23746, #4380 ), #24276, .T. ) ;
#19181=ORIENTED_EDGE ( 'NONE', *, *, #18189, .F. ) ;
#19214=CARTESIAN_POINT ( 'NONE',  ( -0.3759206409296168561, 0.2989751379763687655, 0.2362204724409447676 ) ) ;
#19220=CARTESIAN_POINT ( 'NONE',  ( 0.000000000000000000, 0.000000000000000000, 0.02362204724409448786 ) ) ;
#19223=DIRECTION ( 'NONE',  ( 0.000000000000000000, 0.000000000000000000, 1.000000000000000000 ) ) ;
#19248=CYLINDRICAL_SURFACE ( 'NONE', #17512, 0.6881889763779527325 ) ;
#19250=DIRECTION ( 'NONE',  ( 0.000000000000000000, 0.000000000000000000, 1.000000000000000000 ) ) ;
#19259=DIRECTION ( 'NONE',  ( -0.7818314824680298036, 0.6234898018587337054, 0.000000000000000000 ) ) ;
#19260=CARTESIAN_POINT ( 'NONE',  ( -0.2228021814315760130, -0.4641672719513419976, 0.1473214333387365127 ) ) ;
#19266=AXIS2_PLACEMENT_3D ( 'NONE', #4031, #14217, #1347 ) ;
#19269=EDGE_CURVE ( 'NONE', #25742, #11937, #1016, .T. ) ;
#19272=DIRECTION ( 'NONE',  ( 0.000000000000000000, 1.000000000000000000, 0.000000000000000000 ) ) ;
#19286=CARTESIAN_POINT ( 'NONE',  ( 0.8031496062992127261, 0.000000000000000000, 0.4724409448818898127 ) ) ;
#19347=ORIENTED_EDGE ( 'NONE', *, *, #209, .F. ) ;
#19356=B_SPLINE_CURVE_WITH_KNOTS ( 'NONE', 3,
 ( #19869, #21719, #11248, #21581, #9115, #26224 ),
 .UNSPECIFIED., .F., .F.,
 ( 4, 2, 4 ),
 ( 1.217380381967464009, 1.219305002860850085, 1.221229623754231941 ),
 .UNSPECIFIED. ) ;
#19364=CIRCLE ( 'NONE', #9878, 0.5322834645669292097 ) ;
#19366=CARTESIAN_POINT ( 'NONE',  ( 0.000000000000000000, 0.5322834645669292097, 0.4062992125984251635 ) ) ;
#19373=CARTESIAN_POINT ( 'NONE',  ( -0.4771018889076559244, 0.3804760601893846794, 0.1062972440944881941 ) ) ;
#19384=VERTEX_POINT ( 'NONE', #16487 ) ;
#19403=FACE_OUTER_BOUND ( 'NONE', #1069, .T. ) ;
#19412=CARTESIAN_POINT ( 'NONE',  ( -0.5501272682971083405, 0.4396946356847500903, 0.1443310008616609796 ) ) ;
#19428=CYLINDRICAL_SURFACE ( 'NONE', #6272, 0.6881889763779527325 ) ;
#19443=ORIENTED_EDGE ( 'NONE', *, *, #26237, .T. ) ;
#19445=DIRECTION ( 'NONE',  ( 0.000000000000000000, 1.000000000000000000, 0.000000000000000000 ) ) ;
#19490=CARTESIAN_POINT ( 'NONE',  ( 0.0007756954652683944150, 0.7174612052770362736, 0.1601585119462015649 ) ) ;
#19502=ORIENTED_EDGE ( 'NONE', *, *, #21044, .T. ) ;
#19539=VERTEX_POINT ( 'NONE', #6017 ) ;
#19543=CARTESIAN_POINT ( 'NONE',  ( -0.4771018889076559244, 0.3804760601893846794, 0.2362204724409449064 ) ) ;
#19568=ORIENTED_EDGE ( 'NONE', *, *, #11269, .F. ) ;
#19570=ORIENTED_EDGE ( 'NONE', *, *, #25984, .T. ) ;
#19574=CARTESIAN_POINT ( 'NONE',  ( 0.5188388941967637669, -0.1188778293835250077, 0.1322818204150990051 ) ) ;
#19581=DIRECTION ( 'NONE',  ( 0.000000000000000000, 1.000000000000000000, 0.000000000000000000 ) ) ;
#19588=EDGE_CURVE ( 'NONE', #16922, #24495, #3701, .T. ) ;
#19607=AXIS2_PLACEMENT_3D ( 'NONE', #3051, #7174, #22282 ) ;
#19609=EDGE_LOOP ( 'NONE', ( #10411, #18672, #21247, #26102 ) ) ;
#19613=ORIENTED_EDGE ( 'NONE', *, *, #20639, .T. ) ;
#19620=AXIS2_PLACEMENT_3D ( 'NONE', #7961, #9924, #1874 ) ;
#19624=ORIENTED_EDGE ( 'NONE', *, *, #18240, .F. ) ;
#19632=EDGE_CURVE ( 'NONE', #5702, #13442, #3384, .T. ) ;
#19664=EDGE_CURVE ( 'NONE', #13442, #4356, #8837, .T. ) ;
#19667=CARTESIAN_POINT ( 'NONE',  ( -0.4716287720758560176, -0.1069935333117274234, 0.2715646632661209425 ) ) ;
#19671=DIRECTION ( 'NONE',  ( 0.000000000000000000, -1.000000000000000000, 0.000000000000000000 ) ) ;
#19672=DIRECTION ( 'NONE',  ( 0.000000000000000000, 0.000000000000000000, 1.000000000000000000 ) ) ;
#19681=DIRECTION ( 'NONE',  ( 0.000000000000000000, 0.000000000000000000, -1.000000000000000000 ) ) ;
#19683=EDGE_CURVE ( 'NONE', #23783, #23531, #7029, .T. ) ;
#19697=DIRECTION ( 'NONE',  ( -0.9009688679024191460, 0.4338837391175580094, 0.000000000000000000 ) ) ;
#19700=FACE_OUTER_BOUND ( 'NONE', #20375, .T. ) ;
#19707=CARTESIAN_POINT ( 'NONE',  ( 0.5187889641967551313, -0.1190953285357214675, 0.1322834645669291320 ) ) ;
#19710=B_SPLINE_CURVE_WITH_KNOTS ( 'NONE', 3,
 ( #18238, #15605, #5413, #902, #2714, #11348 ),
 .UNSPECIFIED., .F., .F.,
 ( 4, 2, 4 ),
 ( 0.3864984308775630262, 0.3881911340211369743, 0.3898838371647120327 ),
 .UNSPECIFIED. ) ;
#19735=CARTESIAN_POINT ( 'NONE',  ( 0.5099673189336091372, -0.1157175986333315310, 0.1392975274251336271 ) ) ;
#19754=CARTESIAN_POINT ( 'NONE',  ( -0.5190368482393039606, -0.1180105360553399679, 0.3401591244667909186 ) ) ;
#19757=CARTESIAN_POINT ( 'NONE',  ( 0.0006345105826660207057, 0.4803145415259078566, 0.2194422276352448742 ) ) ;
#19779=CARTESIAN_POINT ( 'NONE',  ( 0.3048711895202321220, -0.6348424542973617468, 0.1443310008636820574 ) ) ;
#19780=ADVANCED_FACE ( 'NONE', ( #492, #19700 ), #20531, .T. ) ;
#19798=AXIS2_PLACEMENT_3D ( 'NONE', #6422, #6837, #4301 ) ;
#19801=CARTESIAN_POINT ( 'NONE',  ( 0.4681308612729627727, -0.1074986424507606286, 0.2362204724409450174 ) ) ;
#19804=DIRECTION ( 'NONE',  ( 1.000000000000000000, 0.000000000000000000, 0.000000000000000000 ) ) ;
#19805=CARTESIAN_POINT ( 'NONE',  ( -0.2990496115119744003, -0.6198172806990825956, 0.1322818203437346463 ) ) ;
#19807=DIRECTION ( 'NONE',  ( 0.000000000000000000, -1.000000000000000000, 0.000000000000000000 ) ) ;
#19816=AXIS2_PLACEMENT_3D ( 'NONE', #20319, #14263, #9562 ) ;
#19829=DIRECTION ( 'NONE',  ( 0.000000000000000000, 1.000000000000000000, 0.000000000000000000 ) ) ;
#19859=CARTESIAN_POINT ( 'NONE',  ( -0.4160174684701747894, 0.3320469875258716397, 0.1322810039474933141 ) ) ;
#19865=CIRCLE ( 'NONE', #14486, 0.6881889763779527325 ) ;
#19866=ORIENTED_EDGE ( 'NONE', *, *, #11853, .F. ) ;
#19869=CARTESIAN_POINT ( 'NONE',  ( -0.5385210225480960844, 0.4284847435812472183, 0.3401574803149606252 ) ) ;
#19875=VERTEX_POINT ( 'NONE', #26880 ) ;
#19881=ORIENTED_EDGE ( 'NONE', *, *, #26486, .T. ) ;
#19900=CARTESIAN_POINT ( 'NONE',  ( 0.4084310843282699111, 0.3265597623324891785, 0.1392975274205298652 ) ) ;
#19911=CARTESIAN_POINT ( 'NONE',  ( 0.000000000000000000, 0.5322834645669292097, -1.092739370078740131E-17 ) ) ;
#19942=ORIENTED_EDGE ( 'NONE', *, *, #17530, .F. ) ;
#19944=CARTESIAN_POINT ( 'NONE',  ( 0.7217751814634446594, -0.1639319465208047555, 0.2161412452816648122 ) ) ;
#19948=ORIENTED_EDGE ( 'NONE', *, *, #19664, .F. ) ;
#19953=ORIENTED_EDGE ( 'NONE', *, *, #6623, .F. ) ;
#19957=DIRECTION ( 'NONE',  ( 1.000000000000000000, 0.000000000000000000, 0.000000000000000000 ) ) ;
#19960=B_SPLINE_CURVE_WITH_KNOTS ( 'NONE', 3,
 ( #18167, #22577, #9276, #10271, #23012, #12257, #20879, #22868 ),
 .UNSPECIFIED., .F., .F.,
 ( 4, 2, 2, 4 ),
 ( 0.000000000000000000, 0.1250000000000001388, 0.2500000000000002776, 0.5000000000000000000 ),
 .UNSPECIFIED. ) ;
#19963=CARTESIAN_POINT ( 'NONE',  ( 0.2992781133269515892, -0.6197069291944330427, 0.3401574803149606252 ) ) ;
#19994=CARTESIAN_POINT ( 'NONE',  ( 0.4890020181333677995, -0.1109469068267140701, 0.3080453759527908009 ) ) ;
#20010=EDGE_LOOP ( 'NONE', ( #26031, #18172, #19502, #23090 ) ) ;
#20030=CARTESIAN_POINT ( 'NONE',  ( 0.0006479495459715539770, 0.5014297259271046636, 0.1643955689159069811 ) ) ;
#20048=CARTESIAN_POINT ( 'NONE',  ( -0.5949363243629232079, -0.1357903337134990229, 0.1062972440944881941 ) ) ;
#20068=DIRECTION ( 'NONE',  ( 0.000000000000000000, 0.000000000000000000, 1.000000000000000000 ) ) ;
#20076=CARTESIAN_POINT ( 'NONE',  ( 0.000000000000000000, 0.000000000000000000, 0.2362204724409449064 ) ) ;
#20078=AXIS2_PLACEMENT_3D ( 'NONE', #21852, #9822, #1762 ) ;
#20091=DIRECTION ( 'NONE',  ( 0.000000000000000000, 0.000000000000000000, -1.000000000000000000 ) ) ;
#20102=( CONVERSION_BASED_UNIT ( 'INCH', #16157 ) LENGTH_UNIT ( ) NAMED_UNIT ( #389 ) ) ;
#20104=CARTESIAN_POINT ( 'NONE',  ( 0.000000000000000000, 0.000000000000000000, 0.3401574803149606252 ) ) ;
#20105=AXIS2_PLACEMENT_3D ( 'NONE', #23765, #5370, #12005 ) ;
#20110=CARTESIAN_POINT ( 'NONE',  ( 0.0006362927944354157799, 0.4836123550484514033, 0.2715646632799083582 ) ) ;
#20129=CARTESIAN_POINT ( 'NONE',  ( -0.4162944719209866196, 0.3316996361851582975, 0.1322810039474933141 ) ) ;
#20138=EDGE_LOOP ( 'NONE', ( #4624, #6129, #9247, #16365 ) ) ;
#20150=FACE_OUTER_BOUND ( 'NONE', #5967, .T. ) ;
#20173=EDGE_LOOP ( 'NONE', ( #26085, #3639, #14840, #20312, #5016, #7159, #19347, #8277, #9253, #20912, #12373, #15277 ) ) ;
#20177=AXIS2_PLACEMENT_3D ( 'NONE', #2734, #17847, #1067 ) ;
#20191=CARTESIAN_POINT ( 'NONE',  ( -0.3916295560398582176, 0.3131429078174728931, 0.3080453759636629374 ) ) ;
#20213=CARTESIAN_POINT ( 'NONE',  ( -0.5375739373539409893, 0.4296723508511055556, 0.1322834645669291320 ) ) ;
#20220=ADVANCED_FACE ( 'NONE', ( #15031 ), #19248, .F. ) ;
#20255=EDGE_CURVE ( 'NONE', #17082, #22865, #22489, .T. ) ;
#20274=ORIENTED_EDGE ( 'NONE', *, *, #13765, .F. ) ;
#20282=CARTESIAN_POINT ( 'NONE',  ( 0.5190862322091315262, -0.1177929122753177127, 0.1322834645669291320 ) ) ;
#20288=CARTESIAN_POINT ( 'NONE',  ( 0.000000000000000000, 0.000000000000000000, 0.02362204724409448786 ) ) ;
#20293=CARTESIAN_POINT ( 'NONE',  ( -0.3105958729529787465, -0.6467467715328735212, 0.3122824329333658833 ) ) ;
#20312=ORIENTED_EDGE ( 'NONE', *, *, #25428, .T. ) ;
#20315=CARTESIAN_POINT ( 'NONE',  ( 0.2647715730835492609, -0.5498038367121063086, 0.1062972440944881941 ) ) ;
#20319=CARTESIAN_POINT ( 'NONE',  ( 0.000000000000000000, 0.000000000000000000, 0.2362204724409449064 ) ) ;
#20321=AXIS2_PLACEMENT_3D ( 'NONE', #1094, #7027, #22134 ) ;
#20325=ORIENTED_EDGE ( 'NONE', *, *, #25653, .F. ) ;
#20355=ORIENTED_EDGE ( 'NONE', *, *, #25903, .F. ) ;
#20358=DIRECTION ( 'NONE',  ( 0.000000000000000000, 0.000000000000000000, 1.000000000000000000 ) ) ;
#20363=DIRECTION ( 'NONE',  ( 0.000000000000000000, -1.000000000000000000, 0.000000000000000000 ) ) ;
#20365=ORIENTED_EDGE ( 'NONE', *, *, #8694, .T. ) ;
#20375=EDGE_LOOP ( 'NONE', ( #14247, #25385 ) ) ;
#20379=ORIENTED_EDGE ( 'NONE', *, *, #12493, .T. ) ;
#20416=VECTOR ( 'NONE', #4848, 39.37007874015748143 ) ;
#20441=CARTESIAN_POINT ( 'NONE',  ( 0.5189874374926378708, -0.1182276436463391700, 0.3401599409343964431 ) ) ;
#20443=EDGE_CURVE ( 'NONE', #22315, #25524, #4315, .T. ) ;
#20454=ORIENTED_EDGE ( 'NONE', *, *, #22252, .F. ) ;
#20458=DIRECTION ( 'NONE',  ( 0.2225209339563153921, 0.9749279121818232863, 0.000000000000000000 ) ) ;
#20486=CARTESIAN_POINT ( 'NONE',  ( -0.3751294191746886164, 0.2999672986753446069, 0.2362204724409450174 ) ) ;
#20498=FACE_OUTER_BOUND ( 'NONE', #7972, .T. ) ;
#20517=LINE ( 'NONE', #1307, #219 ) ;
#20531=SPHERICAL_SURFACE ( 'NONE', #23737, 0.1299232283464566984 ) ;
#20532=CARTESIAN_POINT ( 'NONE',  ( 0.000000000000000000, 0.000000000000000000, 0.06614173228346456601 ) ) ;
#20544=CIRCLE ( 'NONE', #16483, 0.1299232283464566984 ) ;
#20550=CARTESIAN_POINT ( 'NONE',  ( -0.0006568023596628692071, 0.5148705051073217964, 0.1473214333214610816 ) ) ;
#20557=ORIENTED_EDGE ( 'NONE', *, *, #23502, .F. ) ;
#20558=CARTESIAN_POINT ( 'NONE',  ( 0.5501272682988856966, 0.4396946356861675120, 0.1443310008633659491 ) ) ;
#20564=B_SPLINE_CURVE_WITH_KNOTS ( 'NONE', 3,
 ( #8963, #4720, #9224, #6584, #13074, #6859, #6076, #15210 ),
 .UNSPECIFIED., .F., .F.,
 ( 4, 2, 2, 4 ),
 ( 0.000000000000000000, 0.1250000000000001943, 0.2500000000000003886, 0.5000000000000000000 ),
 .UNSPECIFIED. ) ;
#20569=DIRECTION ( 'NONE',  ( 0.000000000000000000, 1.000000000000000000, 0.000000000000000000 ) ) ;
#20576=VERTEX_POINT ( 'NONE', #8072 ) ;
#20592=ORIENTED_EDGE ( 'NONE', *, *, #25342, .F. ) ;
#20621=CARTESIAN_POINT ( 'NONE',  ( -0.3759206409296169116, 0.2989751379763687655, 0.2529987172502118908 ) ) ;
#20629=FACE_OUTER_BOUND ( 'NONE', #23640, .T. ) ;
#20639=EDGE_CURVE ( 'NONE', #11291, #2213, #22468, .T. ) ;
#20643=CARTESIAN_POINT ( 'NONE',  ( 0.5382052855068000241, 0.4288813374988101890, 0.3401599409343964431 ) ) ;
#20657=CARTESIAN_POINT ( 'NONE',  ( -0.4157391792961063204, 0.3323952789219086768, 0.3401574803149606252 ) ) ;
#20658=EDGE_CURVE ( 'NONE', #21309, #24096, #27540, .T. ) ;
#20662=CARTESIAN_POINT ( 'NONE',  ( 0.3197948809217066590, -0.6622502000673956557, 0.1960773254355315520 ) ) ;
#20682=CARTESIAN_POINT ( 'NONE',  ( -0.2239856983871502394, -0.4635973202214443978, 0.1473214333416535404 ) ) ;
#20705=CARTESIAN_POINT ( 'NONE',  ( -0.5378903297326614874, 0.4292762795476984805, 0.1322810039474933141 ) ) ;
#20741=ORIENTED_EDGE ( 'NONE', *, *, #8401, .F. ) ;
#20747=EDGE_LOOP ( 'NONE', ( #4352, #13404, #18214, #21432, #26157, #15099 ) ) ;
#20748=ORIENTED_EDGE ( 'NONE', *, *, #15398, .F. ) ;
#20788=ORIENTED_EDGE ( 'NONE', *, *, #14957, .T. ) ;
#20791=EDGE_CURVE ( 'NONE', #6332, #16370, #16183, .T. ) ;
#20808=DIRECTION ( 'NONE',  ( 0.000000000000000000, -1.000000000000000000, 0.000000000000000000 ) ) ;
#20816=ORIENTED_EDGE ( 'NONE', *, *, #22959, .T. ) ;
#20821=VERTEX_POINT ( 'NONE', #7862 ) ;
#20828=ORIENTED_EDGE ( 'NONE', *, *, #4155, .T. ) ;
#20829=CARTESIAN_POINT ( 'NONE',  ( 0.5744851493179060631, 0.4591414886162703546, 0.1960773254404601651 ) ) ;
#20832=EDGE_LOOP ( 'NONE', ( #3306, #5378, #20365, #23809 ) ) ;
#20841=ORIENTED_EDGE ( 'NONE', *, *, #22731, .T. ) ;
#20855=CARTESIAN_POINT ( 'NONE',  ( -0.4771018889076559244, 0.3804760601893846794, 0.2362204724409449064 ) ) ;
#20864=DIRECTION ( 'NONE',  ( 0.000000000000000000, 0.000000000000000000, 1.000000000000000000 ) ) ;
#20879=CARTESIAN_POINT ( 'NONE',  ( 0.3759206409296168561, 0.2989751379763686545, 0.2194422276324867749 ) ) ;
#20891=ADVANCED_FACE ( 'NONE', ( #23814 ), #19428, .F. ) ;
#20909=AXIS2_PLACEMENT_3D ( 'NONE', #18077, #7377, #15851 ) ;
#20912=ORIENTED_EDGE ( 'NONE', *, *, #7229, .F. ) ;
#20917=CARTESIAN_POINT ( 'NONE',  ( -0.3119936278821711650, -0.6460736482326152608, 0.1601585119449864536 ) ) ;
#20949=CARTESIAN_POINT ( 'NONE',  ( -0.0007856387884314780523, 0.7354206117097525919, 0.1960773254409858557 ) ) ;
#20953=CARTESIAN_POINT ( 'NONE',  ( 0.4771018889076559244, 0.3804760601893846794, 0.1062972440944881941 ) ) ;
#20980=CARTESIAN_POINT ( 'NONE',  ( 0.000000000000000000, 0.000000000000000000, 0.4724409448818898127 ) ) ;
#20982=CIRCLE ( 'NONE', #26376, 0.5322834645669292097 ) ;
#20987=DIRECTION ( 'NONE',  ( 0.000000000000000000, 0.000000000000000000, 1.000000000000000000 ) ) ;
#21004=DIRECTION ( 'NONE',  ( 0.000000000000000000, 1.000000000000000000, 0.000000000000000000 ) ) ;
#21006=VERTEX_POINT ( 'NONE', #13611 ) ;
#21035=CARTESIAN_POINT ( 'NONE',  ( -0.3785000865559329797, 0.3010298976870116050, 0.2715646632809148309 ) ) ;
#21044=EDGE_CURVE ( 'NONE', #27874, #401, #15088, .T. ) ;
#21054=EDGE_CURVE ( 'NONE', #21624, #9806, #17955, .T. ) ;
#21059=ORIENTED_EDGE ( 'NONE', *, *, #15121, .F. ) ;
#21076=( CONVERSION_BASED_UNIT ( 'INCH', #19096 ) LENGTH_UNIT ( ) NAMED_UNIT ( #23345 ) ) ;
#21090=CARTESIAN_POINT ( 'NONE',  ( -0.0007756954652701438836, 0.7174612052774099746, 0.1601585119466828466 ) ) ;
#21092=TOROIDAL_SURFACE ( 'NONE', #21557, 0.4173228346456693272, 0.02362204724409448786 ) ;
#21101=CARTESIAN_POINT ( 'NONE',  ( 0.2239856983846744420, -0.4635973202162851914, 0.3251195115343817332 ) ) ;
#21132=ORIENTED_EDGE ( 'NONE', *, *, #19632, .F. ) ;
#21149=ADVANCED_FACE ( 'NONE', ( #19110 ), #12597, .F. ) ;
#21176=DIRECTION ( 'NONE',  ( 0.000000000000000000, -1.000000000000000000, 0.000000000000000000 ) ) ;
#21177=CARTESIAN_POINT ( 'NONE',  ( 0.4803149606299212393, 0.000000000000000000, 0.2362204724409449064 ) ) ;
#21182=AXIS2_PLACEMENT_3D ( 'NONE', #6494, #15125, #23733 ) ;
#21208=VERTEX_POINT ( 'NONE', #20953 ) ;
#21210=CARTESIAN_POINT ( 'NONE',  ( -0.0006679551606482677165, 0.5322830454629158270, 0.3401574803149606252 ) ) ;
#21220=AXIS2_PLACEMENT_3D ( 'NONE', #17810, #19807, #19681 ) ;
#21247=ORIENTED_EDGE ( 'NONE', *, *, #209, .T. ) ;
#21251=EDGE_LOOP ( 'NONE', ( #27057, #26189, #22057, #1291, #11731, #7896 ) ) ;
#21258=VERTEX_POINT ( 'NONE', #8517 ) ;
#21273=VERTEX_POINT ( 'NONE', #17554 ) ;
#21309=VERTEX_POINT ( 'NONE', #22059 ) ;
#21313=DIRECTION ( 'NONE',  ( -0.2225209339563143096, 0.9749279121818237304, 0.000000000000000000 ) ) ;
#21317=EDGE_CURVE ( 'NONE', #25524, #21624, #10358, .T. ) ;
#21319=CARTESIAN_POINT ( 'NONE',  ( 0.000000000000000000, 0.000000000000000000, 0.02362204724409448786 ) ) ;
#21354=ORIENTED_EDGE ( 'NONE', *, *, #4808, .F. ) ;
#21362=AXIS2_PLACEMENT_3D ( 'NONE', #2167, #8795, #26172 ) ;
#21367=AXIS2_PLACEMENT_3D ( 'NONE', #22434, #26809, #7456 ) ;
#21370=CIRCLE ( 'NONE', #9163, 0.4803149606299212393 ) ;
#21379=CARTESIAN_POINT ( 'NONE',  ( -0.0007683673430022958887, 0.7042519390035199001, 0.3281099440177754345 ) ) ;
#21381=CARTESIAN_POINT ( 'NONE',  ( 0.000000000000000000, 0.000000000000000000, 0.2362204724409449064 ) ) ;
#21419=CARTESIAN_POINT ( 'NONE',  ( 0.000000000000000000, 0.000000000000000000, 0.2362204724409449064 ) ) ;
#21426=CARTESIAN_POINT ( 'NONE',  ( 0.000000000000000000, 0.3937007874015748254, 0.2362204724409449064 ) ) ;
#21428=CARTESIAN_POINT ( 'NONE',  ( -0.7171569026236448430, -0.1628805401839451827, 0.1960773254322785986 ) ) ;
#21431=CARTESIAN_POINT ( 'NONE',  ( 0.5377323685532543474, 0.4294741335735771659, 0.1322818203437346463 ) ) ;
#21432=ORIENTED_EDGE ( 'NONE', *, *, #14714, .F. ) ;
#21440=VERTEX_POINT ( 'NONE', #14447 ) ;
#21460=ORIENTED_EDGE ( 'NONE', *, *, #16074, .F. ) ;
#21471=AXIS2_PLACEMENT_3D ( 'NONE', #7198, #22310, #13837 ) ;
#21479=EDGE_CURVE ( 'NONE', #24310, #3886, #9270, .T. ) ;
#21482=DIRECTION ( 'NONE',  ( 0.000000000000000000, 1.000000000000000000, 0.000000000000000000 ) ) ;
#21485=DIRECTION ( 'NONE',  ( 0.7818314824680303587, 0.6234898018587330393, -0.000000000000000000 ) ) ;
#21492=CARTESIAN_POINT ( 'NONE',  ( -0.5099673189325635292, -0.1157175986330993001, 0.1392975274259370122 ) ) ;
#21504=FACE_OUTER_BOUND ( 'NONE', #5498, .T. ) ;
#21522=CARTESIAN_POINT ( 'NONE',  ( 0.7171569026264477120, -0.1628805401845836165, 0.2763636194414290093 ) ) ;
#21524=ORIENTED_EDGE ( 'NONE', *, *, #22466, .F. ) ;
#21557=AXIS2_PLACEMENT_3D ( 'NONE', #24443, #24589, #1017 ) ;
#21580=ORIENTED_EDGE ( 'NONE', *, *, #19588, .T. ) ;
#21581=CARTESIAN_POINT ( 'NONE',  ( -0.5378903297326614874, 0.4292762795476984805, 0.3401599409343964431 ) ) ;
#21582=SHAPE_REPRESENTATION_RELATIONSHIP ( 'NONE' , 'NONE' ,  #15008, #16079 ) ;
#21591=EDGE_LOOP ( 'NONE', ( #432, #23578, #6620, #27778 ) ) ;
#21604=ADVANCED_FACE ( 'NONE', ( #21903 ), #1426, .T. ) ;
#21605=CIRCLE ( 'NONE', #26093, 0.02362204724409448092 ) ;
#21607=AXIS2_PLACEMENT_3D ( 'NONE', #10183, #13992, #5373 ) ;
#21609=EDGE_CURVE ( 'NONE', #10683, #25047, #15861, .T. ) ;
#21612=CARTESIAN_POINT ( 'NONE',  ( 0.0006362927944363831051, 0.4836123550491836509, 0.2008762815993576367 ) ) ;
#21620=CARTESIAN_POINT ( 'NONE',  ( -0.4165721057576322606, 0.3313508221749649763, 0.1322834645669291320 ) ) ;
#21623=DIRECTION ( 'NONE',  ( -0.6234898018587330393, 0.7818314824680302477, 0.000000000000000000 ) ) ;
#21624=VERTEX_POINT ( 'NONE', #2131 ) ;
#21641=DIRECTION ( 'NONE',  ( 0.9009688679024191460, 0.4338837391175580094, 0.000000000000000000 ) ) ;
#21655=VERTEX_POINT ( 'NONE', #20048 ) ;
#21659=CARTESIAN_POINT ( 'NONE',  ( 0.0007595033562148819414, 0.6881885572739390167, 0.3401574803149606252 ) ) ;
#21667=DIRECTION ( 'NONE',  ( 0.000000000000000000, 1.000000000000000000, 0.000000000000000000 ) ) ;
#21675=EDGE_CURVE ( 'NONE', #23587, #22315, #26209, .T. ) ;
#21681=VERTEX_POINT ( 'NONE', #13407 ) ;
#21686=VERTEX_POINT ( 'NONE', #699 ) ;
#21687=CARTESIAN_POINT ( 'NONE',  ( 0.4157391792961063204, 0.3323952789219082882, 0.3401574803149606252 ) ) ;
#21704=ORIENTED_EDGE ( 'NONE', *, *, #26242, .F. ) ;
#21710=DIRECTION ( 'NONE',  ( 0.000000000000000000, -1.000000000000000000, 0.000000000000000000 ) ) ;
#21719=CARTESIAN_POINT ( 'NONE',  ( -0.5383630292499967940, 0.4286833100733393742, 0.3401591245381555551 ) ) ;
#21741=CARTESIAN_POINT ( 'NONE',  ( -0.0006479495459697725245, 0.5014297259258653217, 0.3080453759641655909 ) ) ;
#21774=ORIENTED_EDGE ( 'NONE', *, *, #26156, .T. ) ;
#21777=DIRECTION ( 'NONE',  ( 1.000000000000000000, 0.000000000000000000, 0.000000000000000000 ) ) ;
#21781=ORIENTED_EDGE ( 'NONE', *, *, #14553, .F. ) ;
#21790=EDGE_LOOP ( 'NONE', ( #11285, #25893, #16591, #24939, #16449 ) ) ;
#21795=B_SPLINE_CURVE_WITH_KNOTS ( 'NONE', 3,
 ( #4446, #618, #23936, #6704 ),
 .UNSPECIFIED., .F., .F.,
 ( 4, 4 ),
 ( 1.217380381967462011, 1.219305002860847864 ),
 .UNSPECIFIED. ) ;
#21799=CYLINDRICAL_SURFACE ( 'NONE', #21362, 0.3937007874015748254 ) ;
#21807=AXIS2_PLACEMENT_3D ( 'NONE', #24291, #18191, #11301 ) ;
#21810=CARTESIAN_POINT ( 'NONE',  ( -0.0006362927944366116549, 0.4836123550488269363, 0.2008762816006358365 ) ) ;
#21820=CARTESIAN_POINT ( 'NONE',  ( 0.4160174684701755665, 0.3320469875258716397, 0.3401599409343964431 ) ) ;
#21841=AXIS2_PLACEMENT_3D ( 'NONE', #27304, #16422, #14314 ) ;
#21846=CARTESIAN_POINT ( 'NONE',  ( 0.5190862322091315262, -0.1177929122753177127, 0.3401574803149606252 ) ) ;
#21852=CARTESIAN_POINT ( 'NONE',  ( 0.000000000000000000, 0.000000000000000000, 0.2362204724409449064 ) ) ;
#21869=B_SPLINE_CURVE_WITH_KNOTS ( 'NONE', 3,
 ( #16331, #13926, #20705, #14221, #12364, #10101 ),
 .UNSPECIFIED., .F., .F.,
 ( 4, 2, 4 ),
 ( 0.4045103800602309896, 0.4064350009536160102, 0.4083596218470010308 ),
 .UNSPECIFIED. ) ;
#21878=CARTESIAN_POINT ( 'NONE',  ( -0.0006345105826668660581, 0.4803145415259079121, 0.2362204724409446843 ) ) ;
#21883=SURFACE_STYLE_FILL_AREA ( #4632 ) ;
#21885=FACE_BOUND ( 'NONE', #2364, .T. ) ;
#21891=B_SPLINE_CURVE_WITH_KNOTS ( 'NONE', 3,
 ( #4533, #2538, #570, #8899, #11161, #4660, #23897, #4792, #19779, #15427 ),
 .UNSPECIFIED., .F., .F.,
 ( 4, 2, 2, 2, 4 ),
 ( 0.000000000000000000, 0.2499999999999996669, 0.4999999999999997780, 0.7499999999999998890, 1.000000000000000000 ),
 .UNSPECIFIED. ) ;
#21903=FACE_OUTER_BOUND ( 'NONE', #25613, .T. ) ;
#21910=CARTESIAN_POINT ( 'NONE',  ( 0.000000000000000000, 0.6102362204724409711, 0.4724409448818898127 ) ) ;
#21931=CARTESIAN_POINT ( 'NONE',  ( 0.5018154743079163982, -0.1152098006149074177, 0.1473214333276229582 ) ) ;
#21936=AXIS2_PLACEMENT_3D ( 'NONE', #26052, #17299, #13383 ) ;
#21946=B_SPLINE_CURVE_WITH_KNOTS ( 'NONE', 3,
 ( #18941, #1712, #3682, #10175 ),
 .UNSPECIFIED., .F., .F.,
 ( 4, 4 ),
 ( 0.3881911340211371408, 0.3898838371647120327 ),
 .UNSPECIFIED. ) ;
#21951=CARTESIAN_POINT ( 'NONE',  ( -0.5614173959463371055, 0.4467232815834303872, 0.1601585119451258976 ) ) ;
#21953=ADVANCED_FACE ( 'NONE', ( #17986, #26622 ), #15896, .T. ) ;
#21956=CARTESIAN_POINT ( 'NONE',  ( -0.4771018889076559244, 0.3804760601893846794, 0.2362204724409449064 ) ) ;
#21961=CARTESIAN_POINT ( 'NONE',  ( 0.4162944719209866196, 0.3316996361851579089, 0.3401599409343964431 ) ) ;
#21969=DIRECTION ( 'NONE',  ( 0.000000000000000000, 0.000000000000000000, -1.000000000000000000 ) ) ;
#21972=CARTESIAN_POINT ( 'NONE',  ( 0.0007595033562148819414, 0.6881885572739390167, 0.1322834645669291320 ) ) ;
#21976=ADVANCED_FACE ( 'NONE', ( #8407 ), #9802, .T. ) ;
#21988=CARTESIAN_POINT ( 'NONE',  ( 0.5614173959472870123, 0.4467232815841902793, 0.3122824329351960304 ) ) ;
#22026=ORIENTED_EDGE ( 'NONE', *, *, #21054, .T. ) ;
#22045=CARTESIAN_POINT ( 'NONE',  ( 0.000000000000000000, 0.000000000000000000, 0.1322834645669291320 ) ) ;
#22052=CARTESIAN_POINT ( 'NONE',  ( 0.000000000000000000, 0.6881889763779527325, 0.4062992125984251635 ) ) ;
#22057=ORIENTED_EDGE ( 'NONE', *, *, #13358, .F. ) ;
#22059=CARTESIAN_POINT ( 'NONE',  ( 0.0007595033562148819414, 0.6881885572739390167, 0.3401574803149606252 ) ) ;
#22061=CARTESIAN_POINT ( 'NONE',  ( 0.6867658503616472787, -0.1559616964381364546, 0.1443310008642350595 ) ) ;
#22063=CARTESIAN_POINT ( 'NONE',  ( 0.000000000000000000, 0.000000000000000000, 0.3401574803149606252 ) ) ;
#22064=CARTESIAN_POINT ( 'NONE',  ( -0.5190862322091315262, -0.1177929122753175184, 0.1322834645669291320 ) ) ;
#22075=CARTESIAN_POINT ( 'NONE',  ( -0.5791695622050556658, 0.4608640948048334796, 0.2161412452746097335 ) ) ;
#22077=CARTESIAN_POINT ( 'NONE',  ( 0.2303471512294322787, -0.4798602677570401598, 0.3401574803149606252 ) ) ;
#22084=FACE_OUTER_BOUND ( 'NONE', #17277, .T. ) ;
#22088=VERTEX_POINT ( 'NONE', #4703 ) ;
#22095=VECTOR ( 'NONE', #17047, 39.37007874015748143 ) ;
#22134=DIRECTION ( 'NONE',  ( 0.000000000000000000, 1.000000000000000000, 0.000000000000000000 ) ) ;
#22152=CARTESIAN_POINT ( 'NONE',  ( 0.3777066424207166095, 0.3020248451656780131, 0.2008762815943767877 ) ) ;
#22165=ORIENTED_EDGE ( 'NONE', *, *, #3806, .T. ) ;
#22180=DIRECTION ( 'NONE',  ( 0.000000000000000000, -1.000000000000000000, 0.000000000000000000 ) ) ;
#22181=AXIS2_PLACEMENT_3D ( 'NONE', #19220, #6374, #15003 ) ;
#22185=FACE_OUTER_BOUND ( 'NONE', #23824, .T. ) ;
#22207=AXIS2_PLACEMENT_3D ( 'NONE', #7117, #15740, #9351 ) ;
#22222=DIRECTION ( 'NONE',  ( 0.6234898018587331503, -0.7818314824680301367, 0.000000000000000000 ) ) ;
#22227=AXIS2_PLACEMENT_3D ( 'NONE', #6889, #410, #24246 ) ;
#22232=CARTESIAN_POINT ( 'NONE',  ( 0.0006568023596629938904, 0.5148705051067553606, 0.3251195115598493612 ) ) ;
#22249=DIRECTION ( 'NONE',  ( 0.000000000000000000, 1.000000000000000000, 0.000000000000000000 ) ) ;
#22250=AXIS2_PLACEMENT_3D ( 'NONE', #9418, #7609, #20458 ) ;
#22252=EDGE_CURVE ( 'NONE', #16370, #27302, #26060, .T. ) ;
#22258=APPLICATION_CONTEXT ( 'automotive_design' ) ;
#22262=DIRECTION ( 'NONE',  ( 1.000000000000000000, 0.000000000000000000, 0.000000000000000000 ) ) ;
#22282=DIRECTION ( 'NONE',  ( 0.000000000000000000, -1.000000000000000000, 0.000000000000000000 ) ) ;
#22284=EDGE_CURVE ( 'NONE', #16925, #16922, #19710, .T. ) ;
#22310=DIRECTION ( 'NONE',  ( 0.000000000000000000, 0.000000000000000000, 1.000000000000000000 ) ) ;
#22313=ORIENTED_EDGE ( 'NONE', *, *, #26242, .T. ) ;
#22315=VERTEX_POINT ( 'NONE', #25849 ) ;
#22321=DIRECTION ( 'NONE',  ( 0.000000000000000000, 0.000000000000000000, 1.000000000000000000 ) ) ;
#22342=B_SPLINE_CURVE_WITH_KNOTS ( 'NONE', 3,
 ( #25009, #8074, #5958, #5672, #14293, #22908 ),
 .UNSPECIFIED., .F., .F.,
 ( 4, 2, 4 ),
 ( 1.217380381967464009, 1.219305002860850085, 1.221229623754233939 ),
 .UNSPECIFIED. ) ;
#22347=CIRCLE ( 'NONE', #11995, 0.5322834645669292097 ) ;
#22348=CARTESIAN_POINT ( 'NONE',  ( -0.5187889641967551313, -0.1190953285357212593, 0.3401574803149606252 ) ) ;
#22354=CARTESIAN_POINT ( 'NONE',  ( 0.5385210225480960844, 0.4284847435812472183, 0.1322834645669291320 ) ) ;
#22377=DIRECTION ( 'NONE',  ( 0.000000000000000000, -1.000000000000000000, 0.000000000000000000 ) ) ;
#22379=B_SPLINE_CURVE_WITH_KNOTS ( 'NONE', 3,
 ( #25465, #7956, #25170, #5411, #17951, #5114, #18083, #899 ),
 .UNSPECIFIED., .F., .F.,
 ( 4, 2, 2, 4 ),
 ( 0.5000000000000000000, 0.7499999999999997780, 0.8749999999999997780, 1.000000000000000000 ),
 .UNSPECIFIED. ) ;
#22407=ORIENTED_EDGE ( 'NONE', *, *, #10935, .T. ) ;
#22420=EDGE_CURVE ( 'NONE', #10381, #4492, #8892, .T. ) ;
#22425=CARTESIAN_POINT ( 'NONE',  ( -0.7214243740405492655, -0.1654689342657525153, 0.2562996995995516225 ) ) ;
#22433=VERTEX_POINT ( 'NONE', #27697 ) ;
#22434=CARTESIAN_POINT ( 'NONE',  ( 0.000000000000000000, 0.000000000000000000, 0.2362204724409449064 ) ) ;
#22438=ORIENTED_EDGE ( 'NONE', *, *, #12493, .F. ) ;
#22454=CARTESIAN_POINT ( 'NONE',  ( -0.3751294191746886164, 0.2999672986753446069, 0.2362204724409450174 ) ) ;
#22466=EDGE_CURVE ( 'NONE', #18057, #18836, #18328, .T. ) ;
#22468=B_SPLINE_CURVE_WITH_KNOTS ( 'NONE', 3,
 ( #19214, #14999, #6650, #23481, #15276, #8353, #4525, #21620 ),
 .UNSPECIFIED., .F., .F.,
 ( 4, 2, 2, 4 ),
 ( 0.5000000000000000000, 0.7500000000000000000, 0.8750000000000001110, 1.000000000000000000 ),
 .UNSPECIFIED. ) ;
#22472=DIRECTION ( 'NONE',  ( 0.000000000000000000, 0.000000000000000000, 1.000000000000000000 ) ) ;
#22477=ORIENTED_EDGE ( 'NONE', *, *, #10981, .T. ) ;
#22489=CIRCLE ( 'NONE', #5329, 0.8267716535433071723 ) ;
#22492=CARTESIAN_POINT ( 'NONE',  ( -0.4834654033843718834, -0.1110087727128845347, 0.2989974301282019020 ) ) ;
#22498=AXIS2_PLACEMENT_3D ( 'NONE', #11963, #7868, #25090 ) ;
#22504=DIRECTION ( 'NONE',  ( 0.000000000000000000, 1.000000000000000000, 0.000000000000000000 ) ) ;
#22505=DIRECTION ( 'NONE',  ( 0.000000000000000000, 0.000000000000000000, 1.000000000000000000 ) ) ;
#22518=CARTESIAN_POINT ( 'NONE',  ( -0.4681308612729627172, -0.1074986424507606841, 0.2362204724409447676 ) ) ;
#22525=CARTESIAN_POINT ( 'NONE',  ( -0.2158067241047623985, -0.4466421405382755561, 0.1734435147819099465 ) ) ;
#22526=ORIENTED_EDGE ( 'NONE', *, *, #12071, .F. ) ;
#22553=CARTESIAN_POINT ( 'NONE',  ( 0.000000000000000000, 0.6102362204724409711, 0.4724409448818898127 ) ) ;
#22566=CARTESIAN_POINT ( 'NONE',  ( -0.6707652279343464530, -0.1538768215239710857, 0.1322834645669291320 ) ) ;
#22569=CARTESIAN_POINT ( 'NONE',  ( 0.000000000000000000, 0.000000000000000000, 0.06614173228346456601 ) ) ;
#22574=ORIENTED_EDGE ( 'NONE', *, *, #7388, .F. ) ;
#22577=CARTESIAN_POINT ( 'NONE',  ( 0.4092566936336781147, 0.3255244810065535677, 0.1392975274217217729 ) ) ;
#22578=CARTESIAN_POINT ( 'NONE',  ( -0.2647715730835492609, -0.5498038367121063086, 0.3661437007874016047 ) ) ;
#22593=DIRECTION ( 'NONE',  ( 0.000000000000000000, 0.000000000000000000, 1.000000000000000000 ) ) ;
#22634=DIRECTION ( 'NONE',  ( 0.000000000000000000, 0.000000000000000000, 1.000000000000000000 ) ) ;
#22651=VERTEX_POINT ( 'NONE', #20315 ) ;
#22659=VERTEX_POINT ( 'NONE', #22578 ) ;
#22690=VERTEX_POINT ( 'NONE', #3488 ) ;
#22702=CARTESIAN_POINT ( 'NONE',  ( 0.5190368482393039606, -0.1180105360553401483, 0.3401591244667909186 ) ) ;
#22712=ADVANCED_FACE ( 'NONE', ( #11838 ), #6485, .F. ) ;
#22714=EDGE_CURVE ( 'NONE', #2281, #2854, #18632, .T. ) ;
#22730=B_SPLINE_CURVE_WITH_KNOTS ( 'NONE', 3,
 ( #17423, #13323, #8671, #2303, #26315, #8808, #10793, #10931, #19412, #15340 ),
 .UNSPECIFIED., .F., .F.,
 ( 4, 2, 2, 2, 4 ),
 ( 0.000000000000000000, 0.2500000000000000000, 0.5000000000000000000, 0.7500000000000000000, 1.000000000000000000 ),
 .UNSPECIFIED. ) ;
#22731=EDGE_CURVE ( 'NONE', #13825, #14265, #9575, .T. ) ;
#22733=CARTESIAN_POINT ( 'NONE',  ( -0.6707652279343347956, -0.1538768215240151616, 0.3401574803149606252 ) ) ;
#22743=DIRECTION ( 'NONE',  ( 1.000000000000000000, 0.000000000000000000, 0.000000000000000000 ) ) ;
#22756=CARTESIAN_POINT ( 'NONE',  ( -0.2089723435111590921, -0.4324731448915377641, 0.2362204724409450174 ) ) ;
#22759=CIRCLE ( 'NONE', #26367, 0.02362204724409448092 ) ;
#22778=B_SPLINE_CURVE_WITH_KNOTS ( 'NONE', 3,
 ( #23626, #27859, #2400, #8495, #4262, #15429 ),
 .UNSPECIFIED., .F., .F.,
 ( 4, 2, 4 ),
 ( 0.4045103800603450095, 0.4064350009536160102, 0.4083596218468860117 ),
 .UNSPECIFIED. ) ;
#22787=B_SPLINE_CURVE_WITH_KNOTS ( 'NONE', 3,
 ( #3582, #20558, #24783, #20829, #7710, #1479, #7412, #12215, #10091, #18700 ),
 .UNSPECIFIED., .F., .F.,
 ( 4, 2, 2, 2, 4 ),
 ( 0.000000000000000000, 0.2500000000000000000, 0.5000000000000000000, 0.7500000000000000000, 1.000000000000000000 ),
 .UNSPECIFIED. ) ;
#22789=EDGE_LOOP ( 'NONE', ( #18824, #14368, #3310, #9642 ) ) ;
#22801=AXIS2_PLACEMENT_3D ( 'NONE', #15799, #26807, #15538 ) ;
#22806=CARTESIAN_POINT ( 'NONE',  ( -0.2181459867477137382, -0.4514914377063456441, 0.1643955689534347675 ) ) ;
#22817=AXIS2_PLACEMENT_3D ( 'NONE', #20980, #18845, #18997 ) ;
#22823=AXIS2_PLACEMENT_3D ( 'NONE', #4575, #2453, #13058 ) ;
#22847=DIRECTION ( 'NONE',  ( 0.000000000000000000, -1.000000000000000000, 0.000000000000000000 ) ) ;
#22865=VERTEX_POINT ( 'NONE', #24108 ) ;
#22868=CARTESIAN_POINT ( 'NONE',  ( 0.3759206409296169116, 0.2989751379763687655, 0.2362204724409450174 ) ) ;
#22883=DIRECTION ( 'NONE',  ( 1.000000000000000000, 0.000000000000000000, 0.000000000000000000 ) ) ;
#22908=CARTESIAN_POINT ( 'NONE',  ( -0.2992781133269515892, -0.6197069291944330427, 0.3401574803149606252 ) ) ;
#22929=ORIENTED_EDGE ( 'NONE', *, *, #13607, .F. ) ;
#22930=ORIENTED_EDGE ( 'NONE', *, *, #19683, .F. ) ;
#22948=EDGE_LOOP ( 'NONE', ( #6199, #5195, #5631, #1449 ) ) ;
#22959=EDGE_CURVE ( 'NONE', #1564, #1942, #19356, .T. ) ;
#22970=EDGE_CURVE ( 'NONE', #401, #1755, #16648, .T. ) ;
#22971=CARTESIAN_POINT ( 'NONE',  ( 0.2078289949484098120, -0.4330237525398076270, 0.2194422276737609812 ) ) ;
#22976=DIRECTION ( 'NONE',  ( 1.224646799147353207E-16, 1.000000000000000000, -0.000000000000000000 ) ) ;
#22995=AXIS2_PLACEMENT_3D ( 'NONE', #16498, #1386, #14406 ) ;
#23001=SPHERICAL_SURFACE ( 'NONE', #4719, 0.1299232283464566984 ) ;
#23012=CARTESIAN_POINT ( 'NONE',  ( 0.3882259019049796867, 0.3087756353516248331, 0.1734435147392032195 ) ) ;
#23028=B_SPLINE_CURVE_WITH_KNOTS ( 'NONE', 3,
 ( #1963, #25699, #14982, #2105, #297, #10572 ),
 .UNSPECIFIED., .F., .F.,
 ( 4, 2, 4 ),
 ( 0.4045103800603460087, 0.4064350009536160102, 0.4083596218468860117 ),
 .UNSPECIFIED. ) ;
#23057=B_SPLINE_CURVE_WITH_KNOTS ( 'NONE', 3,
 ( #18479, #12002, #14572, #10434, #5650, #21035, #20621, #18906 ),
 .UNSPECIFIED., .F., .F.,
 ( 4, 2, 2, 4 ),
 ( 0.000000000000000000, 0.1250000000000000555, 0.2500000000000001110, 0.5000000000000000000 ),
 .UNSPECIFIED. ) ;
#23059=AXIS2_PLACEMENT_3D ( 'NONE', #11500, #13757, #22377 ) ;
#23072=CARTESIAN_POINT ( 'NONE',  ( -0.2305483297598421022, -0.4797636960996590760, 0.3401591244667909186 ) ) ;
#23084=DIRECTION ( 'NONE',  ( 0.000000000000000000, 0.000000000000000000, 1.000000000000000000 ) ) ;
#23090=ORIENTED_EDGE ( 'NONE', *, *, #3378, .F. ) ;
#23116=ORIENTED_EDGE ( 'NONE', *, *, #1068, .F. ) ;
#23134=ADVANCED_FACE ( 'NONE', ( #23270 ), #17257, .F. ) ;
#23140=EDGE_CURVE ( 'NONE', #11663, #20576, #1732, .T. ) ;
#23147=AXIS2_PLACEMENT_3D ( 'NONE', #13319, #2571, #17940 ) ;
#23149=ORIENTED_EDGE ( 'NONE', *, *, #15985, .F. ) ;
#23155=ORIENTED_EDGE ( 'NONE', *, *, #14340, .T. ) ;
#23170=ORIENTED_EDGE ( 'NONE', *, *, #18065, .F. ) ;
#23180=FACE_BOUND ( 'NONE', #8885, .T. ) ;
#23192=TOROIDAL_SURFACE ( 'NONE', #1516, 0.4173228346456693272, 0.02362204724409448786 ) ;
#23216=DIRECTION ( 'NONE',  ( 0.000000000000000000, 0.000000000000000000, 1.000000000000000000 ) ) ;
#23238=ORIENTED_EDGE ( 'NONE', *, *, #21675, .T. ) ;
#23252=B_SPLINE_CURVE_WITH_KNOTS ( 'NONE', 3,
 ( #17114, #21492, #17250, #25194, #7837, #10749, #27191, #1334 ),
 .UNSPECIFIED., .F., .F.,
 ( 4, 2, 2, 4 ),
 ( 0.000000000000000000, 0.1250000000000000833, 0.2500000000000001665, 0.5000000000000000000 ),
 .UNSPECIFIED. ) ;
#23254=VERTEX_POINT ( 'NONE', #1575 ) ;
#23266=CARTESIAN_POINT ( 'NONE',  ( -0.2303471512294322787, -0.4798602677570401598, 0.1322834645669291320 ) ) ;
#23270=FACE_OUTER_BOUND ( 'NONE', #19609, .T. ) ;
#23277=CARTESIAN_POINT ( 'NONE',  ( -0.4173228346456693272, 5.110730736599190647E-17, -5.463696850393700654E-18 ) ) ;
#23286=B_SPLINE_CURVE_WITH_KNOTS ( 'NONE', 3,
 ( #11927, #1063, #20682, #22806, #22525, #15752, #5282, #18258 ),
 .UNSPECIFIED., .F., .F.,
 ( 4, 2, 2, 4 ),
 ( 0.000000000000000000, 0.1250000000000002220, 0.2500000000000002776, 0.5000000000000000000 ),
 .UNSPECIFIED. ) ;
#23287=DIRECTION ( 'NONE',  ( 0.000000000000000000, 0.000000000000000000, 1.000000000000000000 ) ) ;
#23290=ORIENTED_EDGE ( 'NONE', *, *, #26449, .T. ) ;
#23320=ORIENTED_EDGE ( 'NONE', *, *, #4372, .F. ) ;
#23321=ORIENTED_EDGE ( 'NONE', *, *, #22466, .T. ) ;
#23325=DIRECTION ( 'NONE',  ( 0.000000000000000000, 0.000000000000000000, 1.000000000000000000 ) ) ;
#23345=DIMENSIONAL_EXPONENTS ( 1.000000000000000000, 0.000000000000000000, 0.000000000000000000, 0.000000000000000000, 0.000000000000000000, 0.000000000000000000, 0.000000000000000000 ) ;
#23357=ORIENTED_EDGE ( 'NONE', *, *, #15862, .F. ) ;
#23362=CARTESIAN_POINT ( 'NONE',  ( -0.2262947209317479058, -0.4714317853999300256, 0.1392975274300493338 ) ) ;
#23364=CARTESIAN_POINT ( 'NONE',  ( 0.2089723435111824623, -0.4324731448915265508, 0.2362204724409445455 ) ) ;
#23376=EDGE_LOOP ( 'NONE', ( #15957, #7408 ) ) ;
#23392=ORIENTED_EDGE ( 'NONE', *, *, #12085, .F. ) ;
#23413=EDGE_LOOP ( 'NONE', ( #24183, #20454 ) ) ;
#23433=CIRCLE ( 'NONE', #22498, 0.3937007874015748254 ) ;
#23440=CIRCLE ( 'NONE', #15755, 0.6881889763779527325 ) ;
#23455=B_SPLINE_CURVE_WITH_KNOTS ( 'NONE', 3,
 ( #4765, #543, #9139, #21741, #2368, #6492, #11000, #21878 ),
 .UNSPECIFIED., .F., .F.,
 ( 4, 2, 2, 4 ),
 ( 0.000000000000000000, 0.1250000000000001110, 0.2500000000000002220, 0.5000000000000000000 ),
 .UNSPECIFIED. ) ;
#23481=CARTESIAN_POINT ( 'NONE',  ( -0.3882259019063066807, 0.3087756353526792119, 0.1734435147361200746 ) ) ;
#23502=EDGE_CURVE ( 'NONE', #11259, #22433, #15620, .T. ) ;
#23508=EDGE_LOOP ( 'NONE', ( #3571, #4415, #18092, #18203, #20557, #10738 ) ) ;
#23514=ORIENTED_EDGE ( 'NONE', *, *, #18293, .T. ) ;
#23521=FACE_OUTER_BOUND ( 'NONE', #16416, .T. ) ;
#23526=ADVANCED_FACE ( 'NONE', ( #708 ), #9582, .T. ) ;
#23531=VERTEX_POINT ( 'NONE', #11855 ) ;
#23539=CARTESIAN_POINT ( 'NONE',  ( 0.5949363243629232079, -0.1357903337134992172, 0.1062972440944881941 ) ) ;
#23553=CIRCLE ( 'NONE', #8195, 0.3937007874015748254 ) ;
#23562=CARTESIAN_POINT ( 'NONE',  ( -0.7217751814648617481, -0.1639319465211148685, 0.2562996995908388698 ) ) ;
#23565=CARTESIAN_POINT ( 'NONE',  ( 0.5383630292499967940, 0.4286833100733393742, 0.1322818203437346463 ) ) ;
#23573=AXIS2_PLACEMENT_3D ( 'NONE', #6826, #15453, #25899 ) ;
#23578=ORIENTED_EDGE ( 'NONE', *, *, #3674, .F. ) ;
#23587=VERTEX_POINT ( 'NONE', #22733 ) ;
#23604=EDGE_CURVE ( 'NONE', #1421, #11291, #23057, .T. ) ;
#23608=VERTEX_POINT ( 'NONE', #27549 ) ;
#23612=ORIENTED_EDGE ( 'NONE', *, *, #15985, .T. ) ;
#23617=CARTESIAN_POINT ( 'NONE',  ( 0.000000000000000000, 0.6881889763779527325, 0.4724409448818898127 ) ) ;
#23626=CARTESIAN_POINT ( 'NONE',  ( 0.6707652279343464530, -0.1538768215239712522, 0.1322834645669291320 ) ) ;
#23639=B_SPLINE_CURVE_WITH_KNOTS ( 'NONE', 3,
 ( #22756, #16837, #16535, #6110, #25445, #7936, #16693, #5678 ),
 .UNSPECIFIED., .F., .F.,
 ( 4, 2, 2, 4 ),
 ( 0.5000000000000000000, 0.7500000000000003331, 0.8750000000000002220, 1.000000000000000000 ),
 .UNSPECIFIED. ) ;
#23640=EDGE_LOOP ( 'NONE', ( #16937, #13582, #9416, #972 ) ) ;
#23668=CARTESIAN_POINT ( 'NONE',  ( -0.2315507648392299000, -0.4792806379917101678, 0.3401574803149606252 ) ) ;
#23679=ORIENTED_EDGE ( 'NONE', *, *, #18752, .F. ) ;
#23706=ORIENTED_EDGE ( 'NONE', *, *, #2268, .T. ) ;
#23719=EDGE_CURVE ( 'NONE', #3153, #11508, #23028, .T. ) ;
#23731=CARTESIAN_POINT ( 'NONE',  ( -0.5189874374926378708, -0.1182276436463389618, 0.3401599409343964431 ) ) ;
#23733=DIRECTION ( 'NONE',  ( -0.9009688679024190350, 0.4338837391175582314, 0.000000000000000000 ) ) ;
#23736=CARTESIAN_POINT ( 'NONE',  ( 0.0006568023596644008595, 0.5148705051078593664, 0.1473214333209106885 ) ) ;
#23737=AXIS2_PLACEMENT_3D ( 'NONE', #11353, #26452, #22222 ) ;
#23739=ORIENTED_EDGE ( 'NONE', *, *, #86, .T. ) ;
#23746=FACE_OUTER_BOUND ( 'NONE', #9425, .T. ) ;
#23751=ADVANCED_FACE ( 'NONE', ( #6632 ), #4627, .T. ) ;
#23752=CARTESIAN_POINT ( 'NONE',  ( 0.3924375359097452831, 0.3121297331107421580, 0.3080453759670797043 ) ) ;
#23753=ORIENTED_EDGE ( 'NONE', *, *, #9476, .F. ) ;
#23760=DIRECTION ( 'NONE',  ( 1.000000000000000000, 0.000000000000000000, 0.000000000000000000 ) ) ;
#23765=CARTESIAN_POINT ( 'NONE',  ( 0.000000000000000000, 0.000000000000000000, 0.2362204724409449064 ) ) ;
#23766=CARTESIAN_POINT ( 'NONE',  ( 0.2647715730835492609, -0.5498038367121063086, 0.2362204724409449064 ) ) ;
#23772=ADVANCED_FACE ( 'NONE', ( #9005 ), #23192, .T. ) ;
#23782=CARTESIAN_POINT ( 'NONE',  ( 0.5187889641967551313, -0.1190953285357214675, 0.1322834645669291320 ) ) ;
#23783=VERTEX_POINT ( 'NONE', #17083 ) ;
#23804=CARTESIAN_POINT ( 'NONE',  ( -0.6709908451338839619, -0.1528902114222549236, 0.3401599409343967761 ) ) ;
#23809=ORIENTED_EDGE ( 'NONE', *, *, #14629, .F. ) ;
#23814=FACE_OUTER_BOUND ( 'NONE', #27382, .T. ) ;
#23824=EDGE_LOOP ( 'NONE', ( #48, #26959, #18748, #23860 ) ) ;
#23843=CARTESIAN_POINT ( 'NONE',  ( 0.5791695622054565673, 0.4608640948051578867, 0.2562996996039434427 ) ) ;
#23846=EDGE_CURVE ( 'NONE', #17014, #20821, #21370, .T. ) ;
#23860=ORIENTED_EDGE ( 'NONE', *, *, #18502, .F. ) ;
#23874=CARTESIAN_POINT ( 'NONE',  ( -0.5190368482393039606, -0.1180105360553399679, 0.1322818204150990051 ) ) ;
#23881=VERTEX_POINT ( 'NONE', #13803 ) ;
#23886=CARTESIAN_POINT ( 'NONE',  ( 0.0007595033562148819414, 0.6881885572739390167, 0.3401574803149606252 ) ) ;
#23895=CIRCLE ( 'NONE', #2217, 0.5322834645669292097 ) ;
#23897=CARTESIAN_POINT ( 'NONE',  ( 0.3183792087430821205, -0.6629319518596328287, 0.1960773254418380074 ) ) ;
#23923=CARTESIAN_POINT ( 'NONE',  ( 0.7171569026277438974, -0.1628805401848839596, 0.1960773254442478020 ) ) ;
#23928=CARTESIAN_POINT ( 'NONE',  ( 0.2992781133269515892, -0.6197069291944330427, 0.3401574803149606252 ) ) ;
#23936=CARTESIAN_POINT ( 'NONE',  ( -0.0002525749203917906525, 0.6881889763779527325, 0.3401599409343964431 ) ) ;
#23943=ORIENTED_EDGE ( 'NONE', *, *, #1720, .F. ) ;
#23948=DIRECTION ( 'NONE',  ( 0.000000000000000000, 0.000000000000000000, 1.000000000000000000 ) ) ;
#23956=CARTESIAN_POINT ( 'NONE',  ( 0.0002525749203917322682, 0.6881889763779527325, 0.1322810039474933141 ) ) ;
#23963=CARTESIAN_POINT ( 'NONE',  ( -0.4158785340170984557, 0.3322209827720822850, 0.1322818204150988386 ) ) ;
#23966=ORIENTED_EDGE ( 'NONE', *, *, #9320, .T. ) ;
#23981=DIRECTION ( 'NONE',  ( 0.9749279121818237304, 0.2225209339563139488, -0.000000000000000000 ) ) ;
#24001=CARTESIAN_POINT ( 'NONE',  ( 0.3874223757861530171, 0.3097832252395282260, 0.1734435147339651040 ) ) ;
#24003=ORIENTED_EDGE ( 'NONE', *, *, #25984, .F. ) ;
#24016=CARTESIAN_POINT ( 'NONE',  ( 0.2089723435111824623, -0.4324731448915265508, 0.2362204724409445455 ) ) ;
#24038=CARTESIAN_POINT ( 'NONE',  ( 0.000000000000000000, 0.000000000000000000, 0.02362204724409448786 ) ) ;
#24040=CARTESIAN_POINT ( 'NONE',  ( -0.3759206409296168561, 0.2989751379763687655, 0.2362204724409447676 ) ) ;
#24046=CARTESIAN_POINT ( 'NONE',  ( 0.7217751814627907381, -0.1639319465206539039, 0.2562996996045692755 ) ) ;
#24048=ADVANCED_FACE ( 'NONE', ( #7346, #13846 ), #11860, .T. ) ;
#24062=CARTESIAN_POINT ( 'NONE',  ( -0.5754648248623214224, 0.4579130143384639307, 0.1960773254380976105 ) ) ;
#24069=CIRCLE ( 'NONE', #18647, 0.6881889763779527325 ) ;
#24088=CARTESIAN_POINT ( 'NONE',  ( 0.000000000000000000, 0.6881889763779527325, 0.1322810039474933141 ) ) ;
#24096=VERTEX_POINT ( 'NONE', #3088 ) ;
#24097=CARTESIAN_POINT ( 'NONE',  ( 0.000000000000000000, 0.000000000000000000, 0.02362204724409448786 ) ) ;
#24108=CARTESIAN_POINT ( 'NONE',  ( 0.8267716535433071723, 0.000000000000000000, 0.02362204724409448786 ) ) ;
#24110=CARTESIAN_POINT ( 'NONE',  ( 0.4684132450478833976, -0.1062614382955264641, 0.2362204724409446843 ) ) ;
#24120=EDGE_CURVE ( 'NONE', #22088, #15780, #7634, .T. ) ;
#24124=CARTESIAN_POINT ( 'NONE',  ( -0.3183792087428392037, -0.6629319518591524352, 0.1960773254403069543 ) ) ;
#24172=CARTESIAN_POINT ( 'NONE',  ( -0.5018154743035343479, -0.1152098006138999320, 0.1473214333322230285 ) ) ;
#24183=ORIENTED_EDGE ( 'NONE', *, *, #15730, .F. ) ;
#24191=FACE_BOUND ( 'NONE', #2831, .T. ) ;
#24194=B_SPLINE_CURVE_WITH_KNOTS ( 'NONE', 3,
 ( #21846, #17725, #10966, #19994, #2481, #26078, #7274, #15374 ),
 .UNSPECIFIED., .F., .F.,
 ( 4, 2, 2, 4 ),
 ( 0.000000000000000000, 0.1250000000000000000, 0.2500000000000000000, 0.5000000000000000000 ),
 .UNSPECIFIED. ) ;
#24201=CARTESIAN_POINT ( 'NONE',  ( 0.2307489990847578776, -0.4796672131996535526, 0.3401599409343964431 ) ) ;
#24213=DIRECTION ( 'NONE',  ( 0.6234898018587335944, 0.7818314824680296926, 0.000000000000000000 ) ) ;
#24234=CARTESIAN_POINT ( 'NONE',  ( -0.5385210225480960844, 0.4284847435812472183, 0.3401574803149606252 ) ) ;
#24245=ORIENTED_EDGE ( 'NONE', *, *, #20639, .F. ) ;
#24246=DIRECTION ( 'NONE',  ( 0.000000000000000000, 1.000000000000000000, 0.000000000000000000 ) ) ;
#24247=ORIENTED_EDGE ( 'NONE', *, *, #1208, .F. ) ;
#24250=CARTESIAN_POINT ( 'NONE',  ( 0.000000000000000000, 0.000000000000000000, 0.1322834645669291320 ) ) ;
#24251=EDGE_CURVE ( 'NONE', #26228, #11259, #14965, .T. ) ;
#24252=DIRECTION ( 'NONE',  ( 0.000000000000000000, 0.000000000000000000, 1.000000000000000000 ) ) ;
#24253=CARTESIAN_POINT ( 'NONE',  ( -0.3204319178468620910, -0.6672004808830966915, 0.2161412452771441228 ) ) ;
#24256=ORIENTED_EDGE ( 'NONE', *, *, #10601, .T. ) ;
#24259=CARTESIAN_POINT ( 'NONE',  ( -0.5187889641967551313, -0.1190953285357212593, 0.3401574803149606252 ) ) ;
#24260=CARTESIAN_POINT ( 'NONE',  ( -0.2315507648392299000, -0.4792806379917101678, 0.1322834645669291320 ) ) ;
#24273=EDGE_LOOP ( 'NONE', ( #2627, #10550, #19624, #17866, #27736, #24256, #25690, #17303, #15646, #16531, #27258 ) ) ;
#24276=SPHERICAL_SURFACE ( 'NONE', #4368, 0.1299232283464566984 ) ;
#24282=DIRECTION ( 'NONE',  ( 0.000000000000000000, 0.000000000000000000, 1.000000000000000000 ) ) ;
#24290=CIRCLE ( 'NONE', #19798, 0.5322834645669292097 ) ;
#24291=CARTESIAN_POINT ( 'NONE',  ( 0.000000000000000000, 0.000000000000000000, 0.2362204724409449064 ) ) ;
#24310=VERTEX_POINT ( 'NONE', #17776 ) ;
#24311=DIRECTION ( 'NONE',  ( 0.000000000000000000, 0.000000000000000000, 1.000000000000000000 ) ) ;
#24318=DIRECTION ( 'NONE',  ( 0.000000000000000000, -1.000000000000000000, 0.000000000000000000 ) ) ;
#24319=DIRECTION ( 'NONE',  ( 0.000000000000000000, 0.000000000000000000, 1.000000000000000000 ) ) ;
#24327=SPHERICAL_SURFACE ( 'NONE', #1730, 0.1299232283464566984 ) ;
#24381=ORIENTED_EDGE ( 'NONE', *, *, #7891, .F. ) ;
#24382=ORIENTED_EDGE ( 'NONE', *, *, #8243, .F. ) ;
#24392=AXIS2_PLACEMENT_3D ( 'NONE', #24784, #26764, #1211 ) ;
#24406=EDGE_LOOP ( 'NONE', ( #10902, #3557, #6730, #11078 ) ) ;
#24422=B_SPLINE_CURVE_WITH_KNOTS ( 'NONE', 3,
 ( #11821, #14085, #18009, #20441, #22702, #18582 ),
 .UNSPECIFIED., .F., .F.,
 ( 4, 2, 4 ),
 ( 1.162880698919835920, 1.164573402063409979, 1.166266105206986037 ),
 .UNSPECIFIED. ) ;
#24431=CARTESIAN_POINT ( 'NONE',  ( 0.2078289949484099508, -0.4330237525398077936, 0.2362204724409449619 ) ) ;
#24443=CARTESIAN_POINT ( 'NONE',  ( 0.000000000000000000, 0.000000000000000000, 0.4488188976377953110 ) ) ;
#24445=AXIS2_PLACEMENT_3D ( 'NONE', #21419, #14521, #8419 ) ;
#24449=AXIS2_PLACEMENT_3D ( 'NONE', #4985, #6712, #17435 ) ;
#24451=AXIS2_PLACEMENT_3D ( 'NONE', #9165, #1679, #22883 ) ;
#24461=DIRECTION ( 'NONE',  ( 0.000000000000000000, 0.000000000000000000, -1.000000000000000000 ) ) ;
#24486=DIRECTION ( 'NONE',  ( -0.9749279121818237304, -0.2225209339563138378, 0.000000000000000000 ) ) ;
#24495=VERTEX_POINT ( 'NONE', #1452 ) ;
#24520=DIRECTION ( 'NONE',  ( 0.000000000000000000, 0.000000000000000000, 1.000000000000000000 ) ) ;
#24523=CARTESIAN_POINT ( 'NONE',  ( -0.3105958729522376172, -0.6467467715313297560, 0.1601585119463167506 ) ) ;
#24534=DIRECTION ( 'NONE',  ( 1.000000000000000000, 0.000000000000000000, 0.000000000000000000 ) ) ;
#24538=EDGE_CURVE ( 'NONE', #21208, #19384, #14194, .T. ) ;
#24574=CARTESIAN_POINT ( 'NONE',  ( -0.3874223757850451810, 0.3097832252386399365, 0.1734435147365480934 ) ) ;
#24581=DIRECTION ( 'NONE',  ( 0.000000000000000000, 1.000000000000000000, 0.000000000000000000 ) ) ;
#24582=CARTESIAN_POINT ( 'NONE',  ( -0.3197948809234547607, -0.6622502000709752368, 0.2763636194350204134 ) ) ;
#24589=DIRECTION ( 'NONE',  ( 0.000000000000000000, 0.000000000000000000, 1.000000000000000000 ) ) ;
#24599=DIRECTION ( 'NONE',  ( 0.000000000000000000, 0.000000000000000000, 1.000000000000000000 ) ) ;
#24600=CARTESIAN_POINT ( 'NONE',  ( -0.3937007874015748254, 4.966087413865251393E-17, 0.02362204724409448786 ) ) ;
#24605=CARTESIAN_POINT ( 'NONE',  ( 0.2979095355689177493, -0.6203660015065670663, 0.3401574803149606252 ) ) ;
#24667=ORIENTED_EDGE ( 'NONE', *, *, #6377, .F. ) ;
#24680=CARTESIAN_POINT ( 'NONE',  ( 0.6711032387266713251, -0.1523958994812761869, 0.3401574803149606252 ) ) ;
#24701=AXIS2_PLACEMENT_3D ( 'NONE', #4255, #10886, #6936 ) ;
#24707=CARTESIAN_POINT ( 'NONE',  ( 0.2262947209296605477, -0.4714317853956138671, 0.3331434174482444943 ) ) ;
#24723=ORIENTED_EDGE ( 'NONE', *, *, #17291, .T. ) ;
#24735=VERTEX_POINT ( 'NONE', #25834 ) ;
#24749=CIRCLE ( 'NONE', #15317, 0.6881889763779527325 ) ;
#24751=DIRECTION ( 'NONE',  ( 1.000000000000000000, 0.000000000000000000, 0.000000000000000000 ) ) ;
#24752=CARTESIAN_POINT ( 'NONE',  ( 0.6102362204724409711, 0.000000000000000000, 0.2362204724409449064 ) ) ;
#24757=FACE_OUTER_BOUND ( 'NONE', #4150, .T. ) ;
#24758=ORIENTED_EDGE ( 'NONE', *, *, #2752, .T. ) ;
#24765=CARTESIAN_POINT ( 'NONE',  ( 0.2303471512294322787, -0.4798602677570401598, 0.1322834645669291320 ) ) ;
#24778=VERTEX_POINT ( 'NONE', #1680 ) ;
#24783=CARTESIAN_POINT ( 'NONE',  ( 0.5604501195232224342, 0.4479362078551570869, 0.1601585119463994344 ) ) ;
#24784=CARTESIAN_POINT ( 'NONE',  ( 0.000000000000000000, 0.000000000000000000, 0.2362204724409449064 ) ) ;
#24793=CARTESIAN_POINT ( 'NONE',  ( 0.000000000000000000, 0.000000000000000000, 0.4062992125984251635 ) ) ;
#24801=ORIENTED_EDGE ( 'NONE', *, *, #2752, .F. ) ;
#24805=DIRECTION ( 'NONE',  ( 0.000000000000000000, 0.000000000000000000, 1.000000000000000000 ) ) ;
#24813=CARTESIAN_POINT ( 'NONE',  ( 0.000000000000000000, 0.000000000000000000, 0.2362204724409449064 ) ) ;
#24822=FACE_OUTER_BOUND ( 'NONE', #25953, .T. ) ;
#24832=ORIENTED_EDGE ( 'NONE', *, *, #5174, .F. ) ;
#24834=AXIS2_PLACEMENT_3D ( 'NONE', #18003, #24252, #13798 ) ;
#24849=CARTESIAN_POINT ( 'NONE',  ( 0.5096726623840048820, -0.1170085733297153430, 0.3331434174570839235 ) ) ;
#24857=DIRECTION ( 'NONE',  ( -1.000000000000000000, 1.224646799147353454E-16, 0.000000000000000000 ) ) ;
#24887=ORIENTED_EDGE ( 'NONE', *, *, #10585, .T. ) ;
#24926=CIRCLE ( 'NONE', #17703, 0.6881889763779527325 ) ;
#24935=DIRECTION ( 'NONE',  ( -1.000000000000000000, 1.224646799147353454E-16, 0.000000000000000000 ) ) ;
#24939=ORIENTED_EDGE ( 'NONE', *, *, #25653, .T. ) ;
#24942=DIRECTION ( 'NONE',  ( -0.9009688679024190350, -0.4338837391175581759, 0.000000000000000000 ) ) ;
#24948=CIRCLE ( 'NONE', #6014, 0.1299232283464567261 ) ;
#24957=TOROIDAL_SURFACE ( 'NONE', #4206, 0.6102362204724409711, 0.1299212598425196763 ) ;
#24962=CARTESIAN_POINT ( 'NONE',  ( 0.000000000000000000, 0.000000000000000000, -1.092739370078740131E-17 ) ) ;
#24965=ORIENTED_EDGE ( 'NONE', *, *, #25342, .T. ) ;
#24996=CARTESIAN_POINT ( 'NONE',  ( -0.4084310843276608982, 0.3265597623319961840, 0.1392975274211175618 ) ) ;
#25009=CARTESIAN_POINT ( 'NONE',  ( -0.2979095355689177493, -0.6203660015065670663, 0.3401574803149606252 ) ) ;
#25011=CARTESIAN_POINT ( 'NONE',  ( 0.5385210225480960844, 0.4284847435812472183, 0.3401574803149606252 ) ) ;
#25013=CARTESIAN_POINT ( 'NONE',  ( 0.6881889763779527325, 0.000000000000000000, 0.3401574803149606252 ) ) ;
#25021=B_SPLINE_CURVE_WITH_KNOTS ( 'NONE', 3,
 ( #22077, #6979, #24201, #15339, #16771, #10792 ),
 .UNSPECIFIED., .F., .F.,
 ( 4, 2, 4 ),
 ( 1.162880698919837918, 1.164573402063411978, 1.166266105206986037 ),
 .UNSPECIFIED. ) ;
#25025=B_SPLINE_CURVE_WITH_KNOTS ( 'NONE', 3,
 ( #10594, #25860, #6509, #15141, #23752, #13684, #842, #5206 ),
 .UNSPECIFIED., .F., .F.,
 ( 4, 2, 2, 4 ),
 ( 0.5000000000000000000, 0.7500000000000000000, 0.8750000000000000000, 1.000000000000000000 ),
 .UNSPECIFIED. ) ;
#25047=VERTEX_POINT ( 'NONE', #7299 ) ;
#25048=CARTESIAN_POINT ( 'NONE',  ( -0.0007595033562148819414, 0.6881885572739390167, 0.3401574803149606252 ) ) ;
#25068=ORIENTED_EDGE ( 'NONE', *, *, #22731, .F. ) ;
#25070=DIRECTION ( 'NONE',  ( 0.000000000000000000, 0.000000000000000000, 1.000000000000000000 ) ) ;
#25090=DIRECTION ( 'NONE',  ( 0.000000000000000000, -1.000000000000000000, 0.000000000000000000 ) ) ;
#25108=FACE_BOUND ( 'NONE', #26885, .T. ) ;
#25110=VERTEX_POINT ( 'NONE', #3185 ) ;
#25132=B_SPLINE_CURVE_WITH_KNOTS ( 'NONE', 3,
 ( #24431, #16113, #864, #2679, #5224, #11722, #24707, #4803 ),
 .UNSPECIFIED., .F., .F.,
 ( 4, 2, 2, 4 ),
 ( 0.5000000000000000000, 0.7499999999999996669, 0.8749999999999997780, 1.000000000000000000 ),
 .UNSPECIFIED. ) ;
#25149=CARTESIAN_POINT ( 'NONE',  ( -0.4684132450478830645, -0.1062614382955276715, 0.2362204724409449619 ) ) ;
#25163=DIRECTION ( 'NONE',  ( 0.000000000000000000, 0.000000000000000000, 1.000000000000000000 ) ) ;
#25167=ORIENTED_EDGE ( 'NONE', *, *, #12085, .T. ) ;
#25169=CARTESIAN_POINT ( 'NONE',  ( 0.000000000000000000, 0.000000000000000000, 0.1322834645669291320 ) ) ;
#25170=CARTESIAN_POINT ( 'NONE',  ( 0.2104048168823795806, -0.4354435989178285782, 0.2008762816694357189 ) ) ;
#25194=CARTESIAN_POINT ( 'NONE',  ( -0.4890020181310710812, -0.1109469068261995789, 0.1643955689325500014 ) ) ;
#25304=DIRECTION ( 'NONE',  ( 0.000000000000000000, -1.000000000000000000, 0.000000000000000000 ) ) ;
#25342=EDGE_CURVE ( 'NONE', #24096, #5951, #6788, .T. ) ;
#25348=DIRECTION ( 'NONE',  ( 0.000000000000000000, 0.000000000000000000, -1.000000000000000000 ) ) ;
#25367=ORIENTED_EDGE ( 'NONE', *, *, #16658, .T. ) ;
#25379=AXIS2_PLACEMENT_3D ( 'NONE', #20532, #7962, #2989 ) ;
#25380=ORIENTED_EDGE ( 'NONE', *, *, #5920, .T. ) ;
#25385=ORIENTED_EDGE ( 'NONE', *, *, #16581, .T. ) ;
#25412=CARTESIAN_POINT ( 'NONE',  ( 0.000000000000000000, 0.000000000000000000, 0.4488188976377953110 ) ) ;
#25415=AXIS2_PLACEMENT_3D ( 'NONE', #7483, #11859, #9445 ) ;
#25428=EDGE_CURVE ( 'NONE', #21681, #19875, #21946, .T. ) ;
#25431=VERTEX_POINT ( 'NONE', #18221 ) ;
#25433=ORIENTED_EDGE ( 'NONE', *, *, #3674, .T. ) ;
#25444=CARTESIAN_POINT ( 'NONE',  ( 0.5375739373539409893, 0.4296723508511047229, 0.3401574803149606252 ) ) ;
#25445=CARTESIAN_POINT ( 'NONE',  ( -0.2181459867488315385, -0.4514914377086566288, 0.3080453759322188123 ) ) ;
#25465=CARTESIAN_POINT ( 'NONE',  ( 0.2089723435111824623, -0.4324731448915265508, 0.2362204724409445455 ) ) ;
#25524=VERTEX_POINT ( 'NONE', #5826 ) ;
#25534=DIRECTION ( 'NONE',  ( 1.000000000000000000, 0.000000000000000000, 0.000000000000000000 ) ) ;
#25546=ORIENTED_EDGE ( 'NONE', *, *, #6631, .T. ) ;
#25578=VERTEX_POINT ( 'NONE', #26992 ) ;
#25612=CARTESIAN_POINT ( 'NONE',  ( -0.0007856387884325044665, 0.7354206117107146001, 0.2763636194381670075 ) ) ;
#25613=EDGE_LOOP ( 'NONE', ( #12354, #25746, #20379, #107, #4196 ) ) ;
#25635=AXIS2_PLACEMENT_3D ( 'NONE', #18682, #1746, #12196 ) ;
#25639=ORIENTED_EDGE ( 'NONE', *, *, #12047, .T. ) ;
#25640=CARTESIAN_POINT ( 'NONE',  ( -0.6711032387266713251, -0.1523958994812759926, 0.3401574803149606252 ) ) ;
#25653=EDGE_CURVE ( 'NONE', #24735, #27302, #1590, .T. ) ;
#25679=CARTESIAN_POINT ( 'NONE',  ( 0.000000000000000000, 0.000000000000000000, 0.3401574803149606252 ) ) ;
#25690=ORIENTED_EDGE ( 'NONE', *, *, #14743, .T. ) ;
#25699=CARTESIAN_POINT ( 'NONE',  ( -0.6710470464557933834, -0.1526433524318242252, 0.1322818203437344520 ) ) ;
#25716=CIRCLE ( 'NONE', #38, 0.4803149606299212393 ) ;
#25742=VERTEX_POINT ( 'NONE', #8497 ) ;
#25746=ORIENTED_EDGE ( 'NONE', *, *, #8401, .T. ) ;
#25752=EDGE_CURVE ( 'NONE', #14114, #12366, #397, .T. ) ;
#25758=CARTESIAN_POINT ( 'NONE',  ( -0.2988215684304370012, -0.6199272547993012195, 0.1322810039474933141 ) ) ;
#25782=DIRECTION ( 'NONE',  ( 0.000000000000000000, 0.000000000000000000, -1.000000000000000000 ) ) ;
#25785=ORIENTED_EDGE ( 'NONE', *, *, #17291, .F. ) ;
#25804=ADVANCED_FACE ( 'NONE', ( #6940 ), #15562, .F. ) ;
#25834=CARTESIAN_POINT ( 'NONE',  ( 0.8267716535433071723, 0.000000000000000000, 0.4488188976377953110 ) ) ;
#25836=PRODUCT ( 'Deep Groove Ball Bearing 20x42x12', 'Deep Groove Ball Bearing 20x42x12', '', ( #5444 ) ) ;
#25849=CARTESIAN_POINT ( 'NONE',  ( -0.2992781133269515892, -0.6197069291944330427, 0.3401574803149606252 ) ) ;
#25855=CARTESIAN_POINT ( 'NONE',  ( 0.0007683673429997494230, 0.7042519390024098991, 0.1443310008632817665 ) ) ;
#25860=CARTESIAN_POINT ( 'NONE',  ( 0.3759206409296170226, 0.2989751379763687655, 0.2529987172494035375 ) ) ;
#25868=CARTESIAN_POINT ( 'NONE',  ( -0.0005057506112066535546, 0.6881888373222776467, 0.1322818203437346463 ) ) ;
#25893=ORIENTED_EDGE ( 'NONE', *, *, #18319, .T. ) ;
#25898=CARTESIAN_POINT ( 'NONE',  ( 0.0002525749203916739381, 0.6881889763779529545, 0.3401599409343964431 ) ) ;
#25899=DIRECTION ( 'NONE',  ( 1.000000000000000000, 0.000000000000000000, 0.000000000000000000 ) ) ;
#25903=EDGE_CURVE ( 'NONE', #2742, #3153, #26285, .T. ) ;
#25941=ORIENTED_EDGE ( 'NONE', *, *, #6680, .T. ) ;
#25952=ORIENTED_EDGE ( 'NONE', *, *, #4307, .T. ) ;
#25953=EDGE_LOOP ( 'NONE', ( #531, #26281 ) ) ;
#25963=CIRCLE ( 'NONE', #21841, 0.1299232283464566984 ) ;
#25971=EDGE_CURVE ( 'NONE', #9968, #26680, #23252, .T. ) ;
#25973=CARTESIAN_POINT ( 'NONE',  ( -0.2979095355689177493, -0.6203660015065670663, 0.1322834645669291320 ) ) ;
#25979=CARTESIAN_POINT ( 'NONE',  ( -0.3751294191746886164, 0.2999672986753446069, 0.2362204724409450174 ) ) ;
#25984=EDGE_CURVE ( 'NONE', #5951, #9013, #2308, .T. ) ;
#25988=CARTESIAN_POINT ( 'NONE',  ( 0.4157391792961063204, 0.3323952789219082882, 0.1322834645669291320 ) ) ;
#25991=ORIENTED_EDGE ( 'NONE', *, *, #25971, .T. ) ;
#25993=CARTESIAN_POINT ( 'NONE',  ( 0.000000000000000000, 0.6102362204724409711, 0.2362204724409449064 ) ) ;
#26012=FACE_OUTER_BOUND ( 'NONE', #4163, .T. ) ;
#26015=CARTESIAN_POINT ( 'NONE',  ( 0.0006679551606482677165, 0.5322830454629158270, 0.3401574803149606252 ) ) ;
#26027=CARTESIAN_POINT ( 'NONE',  ( 0.4834654033849994370, -0.1110087727130258245, 0.1734435147525180132 ) ) ;
#26031=ORIENTED_EDGE ( 'NONE', *, *, #1526, .T. ) ;
#26037=CARTESIAN_POINT ( 'NONE',  ( 0.2983664441503059428, -0.6201464311010157493, 0.1322810039474933141 ) ) ;
#26051=B_SPLINE_CURVE_WITH_KNOTS ( 'NONE', 3,
 ( #14627, #4140, #14903, #16865 ),
 .UNSPECIFIED., .F., .F.,
 ( 4, 4 ),
 ( 0.3864984308775630262, 0.3881911340211371408 ),
 .UNSPECIFIED. ) ;
#26052=CARTESIAN_POINT ( 'NONE',  ( 0.000000000000000000, 0.000000000000000000, 0.3401574803149606252 ) ) ;
#26060=CIRCLE ( 'NONE', #17490, 0.8031496062992127261 ) ;
#26063=FACE_OUTER_BOUND ( 'NONE', #24273, .T. ) ;
#26071=DIRECTION ( 'NONE',  ( 0.000000000000000000, 0.000000000000000000, 1.000000000000000000 ) ) ;
#26078=CARTESIAN_POINT ( 'NONE',  ( 0.4716287720757130764, -0.1069935333116923404, 0.2715646632655941972 ) ) ;
#26085=ORIENTED_EDGE ( 'NONE', *, *, #24120, .F. ) ;
#26093=AXIS2_PLACEMENT_3D ( 'NONE', #15784, #5037, #4899 ) ;
#26102=ORIENTED_EDGE ( 'NONE', *, *, #15491, .T. ) ;
#26112=CARTESIAN_POINT ( 'NONE',  ( -0.5188885761056504231, -0.1186607836835326668, 0.3401599409343964431 ) ) ;
#26129=CARTESIAN_POINT ( 'NONE',  ( 0.7168072604729537334, -0.1644124225521826632, 0.1960773254416929845 ) ) ;
#26139=CARTESIAN_POINT ( 'NONE',  ( 0.4165721057576322606, 0.3313508221749649763, 0.1322834645669291320 ) ) ;
#26146=DIRECTION ( 'NONE',  ( 0.000000000000000000, 0.000000000000000000, 1.000000000000000000 ) ) ;
#26152=CARTESIAN_POINT ( 'NONE',  ( -0.5099673189338885804, -0.1157175986333887352, 0.3331434174569700146 ) ) ;
#26155=CARTESIAN_POINT ( 'NONE',  ( 0.000000000000000000, 0.000000000000000000, 0.4724409448818898127 ) ) ;
#26156=EDGE_CURVE ( 'NONE', #3371, #21006, #21891, .T. ) ;
#26157=ORIENTED_EDGE ( 'NONE', *, *, #8694, .F. ) ;
#26160=CARTESIAN_POINT ( 'NONE',  ( 0.000000000000000000, 0.000000000000000000, 0.4062992125984251635 ) ) ;
#26172=DIRECTION ( 'NONE',  ( 0.000000000000000000, 1.000000000000000000, 0.000000000000000000 ) ) ;
#26189=ORIENTED_EDGE ( 'NONE', *, *, #6680, .F. ) ;
#26209=CIRCLE ( 'NONE', #9978, 0.6881889763779527325 ) ;
#26224=CARTESIAN_POINT ( 'NONE',  ( -0.5375739373539409893, 0.4296723508511047229, 0.3401574803149606252 ) ) ;
#26228=VERTEX_POINT ( 'NONE', #26532 ) ;
#26233=ORIENTED_EDGE ( 'NONE', *, *, #267, .F. ) ;
#26237=EDGE_CURVE ( 'NONE', #4219, #6332, #14745, .T. ) ;
#26242=EDGE_CURVE ( 'NONE', #21440, #10683, #16105, .T. ) ;
#26257=EDGE_LOOP ( 'NONE', ( #21354, #25380, #11846, #8139 ) ) ;
#26273=CARTESIAN_POINT ( 'NONE',  ( -0.3751294191746890050, 0.2999672986753446069, 0.2529987172464028267 ) ) ;
#26281=ORIENTED_EDGE ( 'NONE', *, *, #22714, .T. ) ;
#26285=B_SPLINE_CURVE_WITH_KNOTS ( 'NONE', 3,
 ( #6188, #4194, #14948, #1928, #23562, #12803, #21428, #14475, #3711, #12723 ),
 .UNSPECIFIED., .F., .F.,
 ( 4, 2, 2, 2, 4 ),
 ( 0.000000000000000000, 0.2500000000000000000, 0.5000000000000000000, 0.7500000000000000000, 1.000000000000000000 ),
 .UNSPECIFIED. ) ;
#26293=DIRECTION ( 'NONE',  ( -0.2225209339563147537, -0.9749279121818235083, 0.000000000000000000 ) ) ;
#26300=ADVANCED_FACE ( 'NONE', ( #991 ), #2946, .F. ) ;
#26315=CARTESIAN_POINT ( 'NONE',  ( -0.5781866216504639722, 0.4620966632784337391, 0.2562996995916987930 ) ) ;
#26326=DIRECTION ( 'NONE',  ( 0.000000000000000000, 0.000000000000000000, 1.000000000000000000 ) ) ;
#26347=CARTESIAN_POINT ( 'NONE',  ( 0.3916295560451238944, 0.3131429078216851902, 0.3080453759735494734 ) ) ;
#26355=CARTESIAN_POINT ( 'NONE',  ( 0.4890020181331002358, -0.1109469068266557973, 0.1643955689295005795 ) ) ;
#26367=AXIS2_PLACEMENT_3D ( 'NONE', #9745, #5226, #24857 ) ;
#26376=AXIS2_PLACEMENT_3D ( 'NONE', #11104, #26478, #22249 ) ;
#26384=ORIENTED_EDGE ( 'NONE', *, *, #11853, .T. ) ;
#26397=CIRCLE ( 'NONE', #15594, 0.1299232283464567261 ) ;
#26398=CARTESIAN_POINT ( 'NONE',  ( -8.427884271297532088E-17, -0.6881889763779527325, 0.4062992125984251635 ) ) ;
#26405=CIRCLE ( 'NONE', #13324, 0.6881889763779527325 ) ;
#26449=EDGE_CURVE ( 'NONE', #17480, #9309, #1161, .T. ) ;
#26452=DIRECTION ( 'NONE',  ( 0.7818314824680300257, 0.6234898018587330393, -0.000000000000000000 ) ) ;
#26453=FACE_OUTER_BOUND ( 'NONE', #5652, .T. ) ;
#26478=DIRECTION ( 'NONE',  ( 0.000000000000000000, 0.000000000000000000, 1.000000000000000000 ) ) ;
#26486=EDGE_CURVE ( 'NONE', #16511, #16609, #874, .T. ) ;
#26488=VERTEX_POINT ( 'NONE', #460 ) ;
#26512=TOROIDAL_SURFACE ( 'NONE', #4866, 0.6102362204724409711, 0.1299212598425196763 ) ;
#26513=DIRECTION ( 'NONE',  ( -0.9009688679024190350, -0.4338837391175581204, 0.000000000000000000 ) ) ;
#26515=AXIS2_PLACEMENT_3D ( 'NONE', #3720, #8251, #18975 ) ;
#26532=CARTESIAN_POINT ( 'NONE',  ( 0.5187889641967551313, -0.1190953285357214675, 0.1322834645669291320 ) ) ;
#26545=AXIS2_PLACEMENT_3D ( 'NONE', #3455, #22976, #24935 ) ;
#26546=CARTESIAN_POINT ( 'NONE',  ( 0.000000000000000000, 0.000000000000000000, 0.2362204724409449064 ) ) ;
#26556=CARTESIAN_POINT ( 'NONE',  ( -0.3062557396312245994, -0.6341756901071494701, 0.3281099440170536230 ) ) ;
#26558=ORIENTED_EDGE ( 'NONE', *, *, #9918, .T. ) ;
#26566=ORIENTED_EDGE ( 'NONE', *, *, #16824, .T. ) ;
#26580=CARTESIAN_POINT ( 'NONE',  ( -0.5510854067052418648, 0.4384931681296231898, 0.3281099440171127424 ) ) ;
#26581=EDGE_CURVE ( 'NONE', #16756, #22088, #14259, .T. ) ;
#26591=ORIENTED_EDGE ( 'NONE', *, *, #15914, .F. ) ;
#26592=CYLINDRICAL_SURFACE ( 'NONE', #22207, 0.8267716535433071723 ) ;
#26601=TOROIDAL_SURFACE ( 'NONE', #18950, 0.6102362204724409711, 0.1299212598425196763 ) ;
#26606=AXIS2_PLACEMENT_3D ( 'NONE', #20076, #24311, #11320 ) ;
#26622=FACE_BOUND ( 'NONE', #17500, .T. ) ;
#26640=AXIS2_PLACEMENT_3D ( 'NONE', #19147, #27780, #8693 ) ;
#26669=CARTESIAN_POINT ( 'NONE',  ( 0.6993003464539847558, -0.1604063846364081614, 0.3122824329341128413 ) ) ;
#26680=VERTEX_POINT ( 'NONE', #25149 ) ;
#26711=ORIENTED_EDGE ( 'NONE', *, *, #20443, .T. ) ;
#26717=CARTESIAN_POINT ( 'NONE',  ( -0.5096726623837302128, -0.1170085733296502145, 0.3331434174568721485 ) ) ;
#26737=ORIENTED_EDGE ( 'NONE', *, *, #26486, .F. ) ;
#26750=CARTESIAN_POINT ( 'NONE',  ( -0.5949363243629232079, -0.1357903337134990229, 0.2362204724409449064 ) ) ;
#26756=CARTESIAN_POINT ( 'NONE',  ( 0.000000000000000000, 0.000000000000000000, 0.1322834645669291320 ) ) ;
#26762=AXIS2_PLACEMENT_3D ( 'NONE', #19543, #19259, #24213 ) ;
#26763=DIRECTION ( 'NONE',  ( 0.000000000000000000, 0.000000000000000000, 1.000000000000000000 ) ) ;
#26764=DIRECTION ( 'NONE',  ( 0.000000000000000000, 0.000000000000000000, 1.000000000000000000 ) ) ;
#26780=CARTESIAN_POINT ( 'NONE',  ( 0.5190862322091315262, -0.1177929122753177127, 0.1322834645669291320 ) ) ;
#26791=AXIS2_PLACEMENT_3D ( 'NONE', #335, #20068, #8912 ) ;
#26807=DIRECTION ( 'NONE',  ( 0.000000000000000000, 0.000000000000000000, -1.000000000000000000 ) ) ;
#26809=DIRECTION ( 'NONE',  ( 0.000000000000000000, 0.000000000000000000, 1.000000000000000000 ) ) ;
#26814=EDGE_CURVE ( 'NONE', #21258, #13999, #2959, .T. ) ;
#26849=CARTESIAN_POINT ( 'NONE',  ( -0.8031496062992127261, 9.980389268641816488E-17, 0.4724409448818898127 ) ) ;
#26876=FACE_OUTER_BOUND ( 'NONE', #20010, .T. ) ;
#26880=CARTESIAN_POINT ( 'NONE',  ( 0.0006679551606482677165, 0.5322830454629158270, 0.1322834645669291320 ) ) ;
#26885=EDGE_LOOP ( 'NONE', ( #23320, #16789, #25068, #25785 ) ) ;
#26901=ORIENTED_EDGE ( 'NONE', *, *, #4307, .F. ) ;
#26904=ADVANCED_FACE ( 'NONE', ( #2252, #12851 ), #1978, .T. ) ;
#26936=FACE_OUTER_BOUND ( 'NONE', #9566, .T. ) ;
#26950=CARTESIAN_POINT ( 'NONE',  ( -0.2307489990847578776, -0.4796672131996535526, 0.1322810039474933141 ) ) ;
#26959=ORIENTED_EDGE ( 'NONE', *, *, #6538, .T. ) ;
#26962=CARTESIAN_POINT ( 'NONE',  ( 0.6708219662590886312, -0.1536294932067318875, 0.3401591245381555551 ) ) ;
#26992=CARTESIAN_POINT ( 'NONE',  ( -0.5187889641967551313, -0.1190953285357212593, 0.3401574803149606252 ) ) ;
#26998=ORIENTED_EDGE ( 'NONE', *, *, #9420, .T. ) ;
#27023=CARTESIAN_POINT ( 'NONE',  ( -0.2307489990847578776, -0.4796672131996535526, 0.3401599409343964431 ) ) ;
#27057=ORIENTED_EDGE ( 'NONE', *, *, #901, .F. ) ;
#27072=AXIS2_PLACEMENT_3D ( 'NONE', #18058, #20358, #16267 ) ;
#27077=VERTEX_POINT ( 'NONE', #2788 ) ;
#27081=EDGE_CURVE ( 'NONE', #14265, #7546, #12724, .T. ) ;
#27095=B_SPLINE_CURVE_WITH_KNOTS ( 'NONE', 3,
 ( #17556, #25898, #223, #21659 ),
 .UNSPECIFIED., .F., .F.,
 ( 4, 4 ),
 ( 1.219305002860847864, 1.221229623754231941 ),
 .UNSPECIFIED. ) ;
#27109=ORIENTED_EDGE ( 'NONE', *, *, #4509, .F. ) ;
#27112=CIRCLE ( 'NONE', #929, 0.5322834645669292097 ) ;
#27186=CARTESIAN_POINT ( 'NONE',  ( -0.8031496062992127261, 9.835745945907876618E-17, 0.02362204724409448786 ) ) ;
#27191=CARTESIAN_POINT ( 'NONE',  ( -0.4684132450478834531, -0.1062614382955279352, 0.2194422276446760245 ) ) ;
#27207=CARTESIAN_POINT ( 'NONE',  ( 0.2078289949484099508, -0.4330237525398077936, 0.2362204724409449619 ) ) ;
#27214=CARTESIAN_POINT ( 'NONE',  ( 0.000000000000000000, 0.5322834645669292097, 0.3401599409343964431 ) ) ;
#27225=FACE_OUTER_BOUND ( 'NONE', #11658, .T. ) ;
#27254=ORIENTED_EDGE ( 'NONE', *, *, #8957, .T. ) ;
#27256=VECTOR ( 'NONE', #23325, 39.37007874015748143 ) ;
#27257=FACE_BOUND ( 'NONE', #1410, .T. ) ;
#27258=ORIENTED_EDGE ( 'NONE', *, *, #14714, .T. ) ;
#27267=EDGE_LOOP ( 'NONE', ( #11703, #6735 ) ) ;
#27276=CARTESIAN_POINT ( 'NONE',  ( -6.518592411209533944E-17, -0.5322834645669292097, 0.4724409448818898127 ) ) ;
#27293=CARTESIAN_POINT ( 'NONE',  ( 0.000000000000000000, 0.000000000000000000, 0.3401574803149606252 ) ) ;
#27298=CARTESIAN_POINT ( 'NONE',  ( -0.2313498293151122209, -0.4793777142568558802, 0.3401591244667909186 ) ) ;
#27301=DIRECTION ( 'NONE',  ( 0.000000000000000000, 0.000000000000000000, 1.000000000000000000 ) ) ;
#27302=VERTEX_POINT ( 'NONE', #19286 ) ;
#27304=CARTESIAN_POINT ( 'NONE',  ( 0.000000000000000000, 0.6102362204724409711, 0.2362204724409449064 ) ) ;
#27306=VERTEX_POINT ( 'NONE', #13069 ) ;
#27307=AXIS2_PLACEMENT_3D ( 'NONE', #26155, #11436, #712 ) ;
#27347=EDGE_CURVE ( 'NONE', #11692, #26228, #11077, .T. ) ;
#27382=EDGE_LOOP ( 'NONE', ( #26233, #24247, #25639, #19570, #25433, #908, #17803, #12464, #12069, #1878, #22026 ) ) ;
#27444=SURFACE_SIDE_STYLE ('',( #21883 ) ) ;
#27448=AXIS2_PLACEMENT_3D ( 'NONE', #12793, #6032, #3604 ) ;
#27453=DIRECTION ( 'NONE',  ( 0.000000000000000000, 1.000000000000000000, 0.000000000000000000 ) ) ;
#27505=CARTESIAN_POINT ( 'NONE',  ( 0.2647715730835492609, -0.5498038367121063086, 0.2362204724409449064 ) ) ;
#27536=ORIENTED_EDGE ( 'NONE', *, *, #23846, .F. ) ;
#27538=AXIS2_PLACEMENT_3D ( 'NONE', #2128, #12715, #12993 ) ;
#27540=B_SPLINE_CURVE_WITH_KNOTS ( 'NONE', 3,
 ( #23886, #17377, #13129, #8480, #12712, #6235, #17100, #19490, #25855, #185 ),
 .UNSPECIFIED., .F., .F.,
 ( 4, 2, 2, 2, 4 ),
 ( 0.000000000000000000, 0.2500000000000000000, 0.5000000000000000000, 0.7500000000000000000, 1.000000000000000000 ),
 .UNSPECIFIED. ) ;
#27549=CARTESIAN_POINT ( 'NONE',  ( 0.4157391792961063204, 0.3323952789219082882, 0.3401574803149606252 ) ) ;
#27559=AXIS2_PLACEMENT_3D ( 'NONE', #27505, #14233, #24942 ) ;
#27560=DIRECTION ( 'NONE',  ( 0.000000000000000000, 0.000000000000000000, 1.000000000000000000 ) ) ;
#27570=ORIENTED_EDGE ( 'NONE', *, *, #14446, .F. ) ;
#27572=CARTESIAN_POINT ( 'NONE',  ( -0.8031496062992127261, 9.980389268641816488E-17, -1.092739370078740131E-17 ) ) ;
#27575=B_SPLINE_CURVE_WITH_KNOTS ( 'NONE', 3,
 ( #11489, #13336, #21961, #21820, #8949, #21687 ),
 .UNSPECIFIED., .F., .F.,
 ( 4, 2, 4 ),
 ( 1.162880698919837918, 1.164573402063411978, 1.166266105206986037 ),
 .UNSPECIFIED. ) ;
#27581=ORIENTED_EDGE ( 'NONE', *, *, #22970, .F. ) ;
#27585=TOROIDAL_SURFACE ( 'NONE', #24392, 0.6102362204724409711, 0.1299212598425196763 ) ;
#27602=VERTEX_POINT ( 'NONE', #6658 ) ;
#27619=ORIENTED_EDGE ( 'NONE', *, *, #4066, .T. ) ;
#27673=VERTEX_POINT ( 'NONE', #15002 ) ;
#27682=B_SPLINE_CURVE_WITH_KNOTS ( 'NONE', 3,
 ( #12481, #2669, #21101, #5998, #6146, #14634, #14777, #24016 ),
 .UNSPECIFIED., .F., .F.,
 ( 4, 2, 2, 4 ),
 ( 0.000000000000000000, 0.1250000000000001943, 0.2500000000000003886, 0.5000000000000000000 ),
 .UNSPECIFIED. ) ;
#27697=CARTESIAN_POINT ( 'NONE',  ( 0.5187889641967551313, -0.1190953285357214675, 0.3401574803149606252 ) ) ;
#27733=DIRECTION ( 'NONE',  ( 1.000000000000000000, 0.000000000000000000, 0.000000000000000000 ) ) ;
#27736=ORIENTED_EDGE ( 'NONE', *, *, #17454, .T. ) ;
#27743=CARTESIAN_POINT ( 'NONE',  ( -0.0007882571242868541359, 0.7401570605733206465, 0.2161412452779228888 ) ) ;
#27752=ORIENTED_EDGE ( 'NONE', *, *, #18240, .T. ) ;
#27766=ORIENTED_EDGE ( 'NONE', *, *, #18319, .F. ) ;
#27778=ORIENTED_EDGE ( 'NONE', *, *, #5174, .T. ) ;
#27780=DIRECTION ( 'NONE',  ( 0.000000000000000000, 0.000000000000000000, 1.000000000000000000 ) ) ;
#27790=B_SPLINE_CURVE_WITH_KNOTS ( 'NONE', 3,
 ( #22354, #23565, #4197, #18078, #21431, #6321 ),
 .UNSPECIFIED., .F., .F.,
 ( 4, 2, 4 ),
 ( 0.4045103800602299904, 0.4064350009536160102, 0.4083596218470010308 ),
 .UNSPECIFIED. ) ;
#27799=EDGE_CURVE ( 'NONE', #24778, #3153, #3941, .T. ) ;
#27830=FACE_BOUND ( 'NONE', #9100, .T. ) ;
#27855=DIRECTION ( 'NONE',  ( 1.000000000000000000, 0.000000000000000000, 0.000000000000000000 ) ) ;
#27858=VERTEX_POINT ( 'NONE', #10831 ) ;
#27859=CARTESIAN_POINT ( 'NONE',  ( 0.6708219662590964028, -0.1536294932067025498, 0.1322818203437344520 ) ) ;
#27874=VERTEX_POINT ( 'NONE', #15059 ) ;
ENDSEC;
END-ISO-10303-21;
